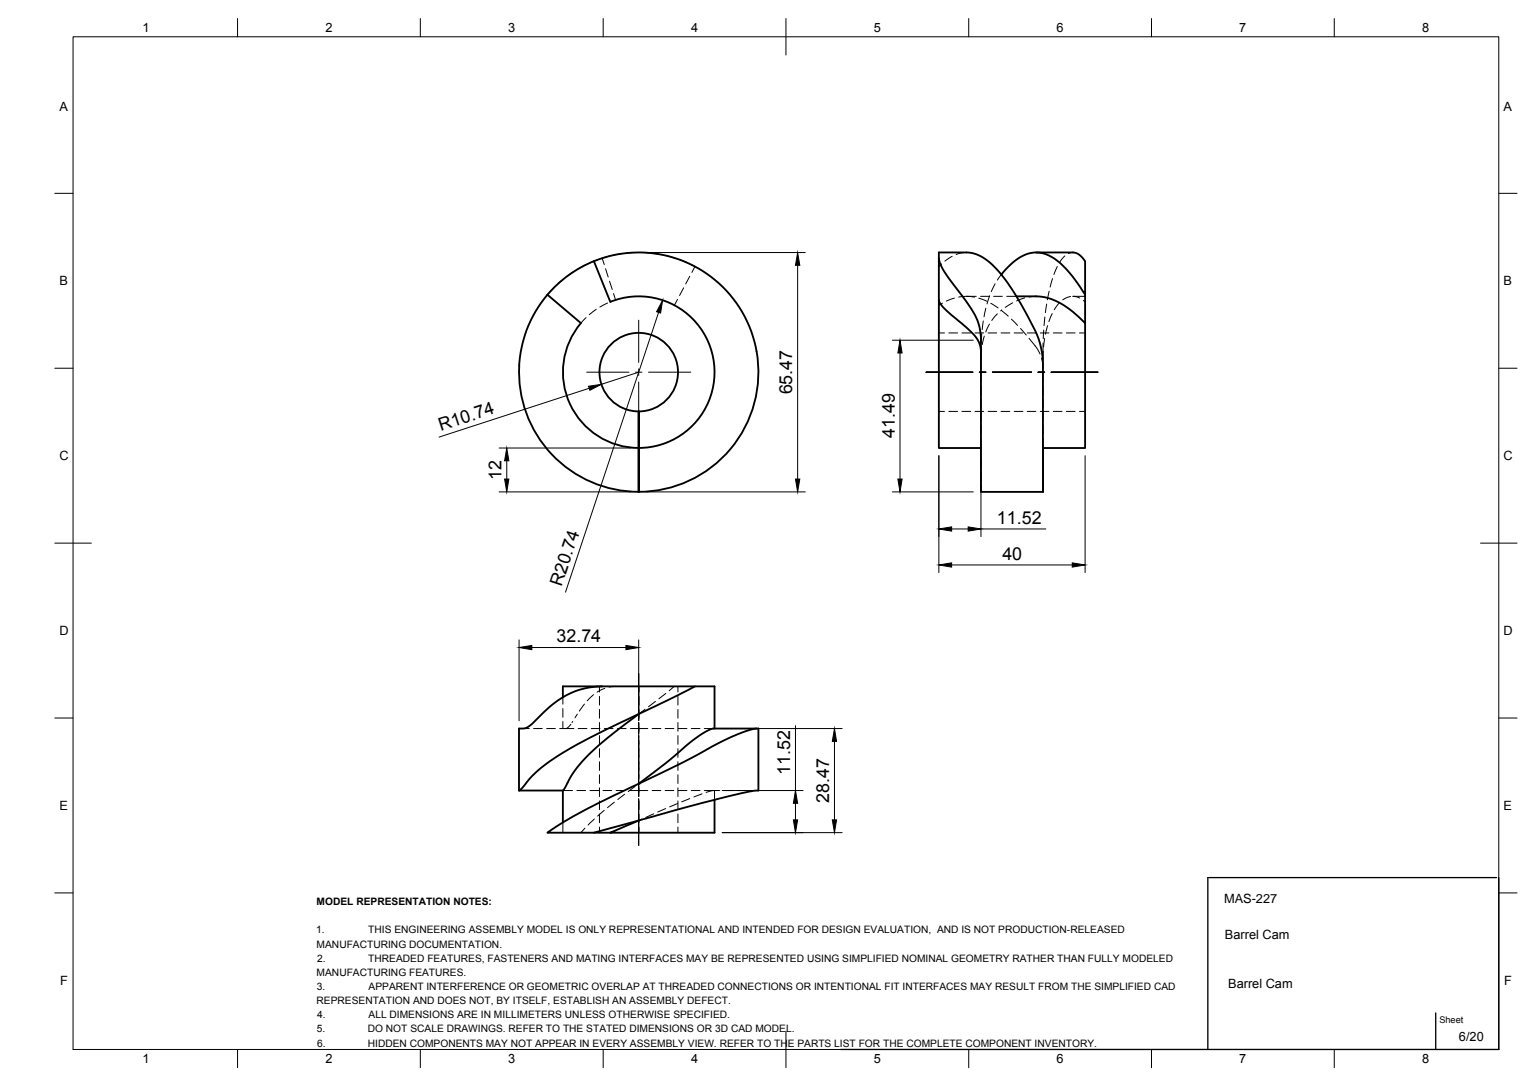
ISO-10303-21;
HEADER;
FILE_DESCRIPTION (('STEP AP214'),
    '1' );
FILE_NAME ( 'Barrel Cam.step', '2026-10-06T08:24:41', ( '' ), ( '' ), 'STEP AP214', 'Unspecified', '' );
FILE_SCHEMA (( 'AUTOMOTIVE_DESIGN' ));
ENDSEC;
DATA;
#20=CARTESIAN_POINT ( 'NONE',  ( 0.3339160553493882300, 0.9180073733179625606, -0.7185233507685039323 ) ) ;
#34=CARTESIAN_POINT ( 'NONE',  ( 0.3976891862754212137, 0.7181140751201200434, -0.6642661073933326943 ) ) ;
#37=ORIENTED_EDGE ( 'NONE', *, *, #10875, .F. ) ;
#42=CARTESIAN_POINT ( 'NONE',  ( -0.3649820351482981340, -1.095990260593795451, -0.3743461065083169559 ) ) ;
#53=DIRECTION ( 'NONE',  ( 0.000000000000000000, 0.000000000000000000, 1.000000000000000000 ) ) ;
#72=CARTESIAN_POINT ( 'NONE',  ( 0.3339160553493882300, 0.7867001919223544082, -0.8344257386302499357 ) ) ;
#75=DIRECTION ( 'NONE',  ( -1.000000000000000000, 0.000000000000000000, 0.000000000000000000 ) ) ;
#104=CARTESIAN_POINT ( 'NONE',  ( -0.6505662911506299162, -0.01797296504513622162, 0.07864818162991654704 ) ) ;
#115=CARTESIAN_POINT ( 'NONE',  ( -0.7432982829791772161, 0.2032415433700952845, -0.2614846436432287091 ) ) ;
#119=CARTESIAN_POINT ( 'NONE',  ( 0.3334645669291338987, -0.9593003268715946108, -0.8847456892490688229 ) ) ;
#171=CARTESIAN_POINT ( 'NONE',  ( -0.3799403784234969272, -1.031940123604548010, -0.2795979895621366063 ) ) ;
#189=ORIENTED_EDGE ( 'NONE', *, *, #329, .F. ) ;
#236=CARTESIAN_POINT ( 'NONE',  ( -0.6370261810203012853, -0.04389326872400071272, -0.2373533611760622331 ) ) ;
#250=CARTESIAN_POINT ( 'NONE',  ( -0.7795729917428700917, 0.3988254141273629982, 0.006455232907575630084 ) ) ;
#260=DIRECTION ( 'NONE',  ( 0.000000000000000000, -0.4702444477782212195, 0.8825362085114445421 ) ) ;
#288=VECTOR ( 'NONE', #25733, 39.37007874015748143 ) ;
#293=CARTESIAN_POINT ( 'NONE',  ( 0.6947676139410623453, 0.7729092381583980709, -0.02125091332446964881 ) ) ;
#329=EDGE_CURVE ( 'NONE', #8378, #18994, #15536, .T. ) ;
#341=B_SPLINE_CURVE_WITH_KNOTS ( 'NONE', 3,
 ( #20281, #13782, #13925, #26772, #18280, #24375, #3448, #26627, #7564, #796, #2888, #16049, #22829 ),
 .UNSPECIFIED., .F., .F.,
 ( 4, 3, 3, 3, 4 ),
 ( 0.01512411120486024073, 0.01814893344583978774, 0.02117375568681436129, 0.02419857792778855668, 0.02712411120487693422 ),
 .UNSPECIFIED. ) ;
#351=CARTESIAN_POINT ( 'NONE',  ( 0.1532705055535415473, -0.8125630895486949390, -0.04838628589907047889 ) ) ;
#357=ORIENTED_EDGE ( 'NONE', *, *, #17696, .F. ) ;
#371=CARTESIAN_POINT ( 'NONE',  ( -0.7635713814939685262, 0.2506761191097937047, -0.2749095812957952911 ) ) ;
#379=CARTESIAN_POINT ( 'NONE',  ( -0.7874015748031496509, 0.8628702403565570167, -0.3208896918748870286 ) ) ;
#411=( GEOMETRIC_REPRESENTATION_CONTEXT ( 3 ) GLOBAL_UNCERTAINTY_ASSIGNED_CONTEXT ( ( #18335 ) ) GLOBAL_UNIT_ASSIGNED_CONTEXT ( ( #27464, #8113, #23091 ) ) REPRESENTATION_CONTEXT ( 'NONE', 'WORKASPACE' ) ) ;
#419=CARTESIAN_POINT ( 'NONE',  ( 0.6015839972843660677, 0.9161431246486984037, -0.1460888818946199375 ) ) ;
#430=DIRECTION ( 'NONE',  ( -1.000000000000000000, 0.000000000000000000, 0.000000000000000000 ) ) ;
#452=CARTESIAN_POINT ( 'NONE',  ( -0.3040421205569480145, 1.249037478091203024, -0.7140903627573721435 ) ) ;
#459=ORIENTED_EDGE ( 'NONE', *, *, #5759, .F. ) ;
#461=DIRECTION ( 'NONE',  ( -1.000000000000000000, 0.000000000000000000, 0.000000000000000000 ) ) ;
#469=CARTESIAN_POINT ( 'NONE',  ( 0.1120675189988346587, -0.7410715175625038897, 0.001857066358701141805 ) ) ;
#483=ADVANCED_FACE ( 'NONE', ( #19377 ), #13015, .T. ) ;
#485=CARTESIAN_POINT ( 'NONE',  ( -0.6370261810203012853, -0.05236013009244417510, -0.08009157605482203346 ) ) ;
#501=CARTESIAN_POINT ( 'NONE',  ( -0.3355349563089153886, 0.1597155962083088576, 0.2362204724409449064 ) ) ;
#527=VERTEX_POINT ( 'NONE', #4408 ) ;
#537=CARTESIAN_POINT ( 'NONE',  ( 0.3843128886798082844, 0.1691648655974895832, -0.07874015748031495954 ) ) ;
#539=CARTESIAN_POINT ( 'NONE',  ( 0.7732217274635454496, 0.5458307047179269400, 0.1151719495065113841 ) ) ;
#550=VERTEX_POINT ( 'NONE', #15439 ) ;
#557=ORIENTED_EDGE ( 'NONE', *, *, #23990, .T. ) ;
#578=EDGE_CURVE ( 'NONE', #17699, #24360, #11458, .T. ) ;
#591=DIRECTION ( 'NONE',  ( 0.000000000000000000, 0.000000000000000000, 1.000000000000000000 ) ) ;
#599=CARTESIAN_POINT ( 'NONE',  ( 0.7872492035923605025, 0.2530564255242896410, -0.2780832379081621952 ) ) ;
#607=VERTEX_POINT ( 'NONE', #866 ) ;
#609=B_SPLINE_CURVE_WITH_KNOTS ( 'NONE', 3,
 ( #16712, #27310, #3855, #5987 ),
 .UNSPECIFIED., .F., .F.,
 ( 4, 4 ),
 ( 0.000000000000000000, 1.000000000000000000 ),
 .UNSPECIFIED. ) ;
#614=APPLICATION_CONTEXT ( 'automotive_design' ) ;
#628=CARTESIAN_POINT ( 'NONE',  ( -0.6633461167951516524, 0.02279600110638677068, 0.07858347093486456325 ) ) ;
#672=CARTESIAN_POINT ( 'NONE',  ( 0.6932508136109228891, 0.7757875710709564165, -0.02341522039927820473 ) ) ;
#686=ORIENTED_EDGE ( 'NONE', *, *, #11935, .F. ) ;
#717=CARTESIAN_POINT ( 'NONE',  ( -0.6562077975700453258, 2.612916929133858441E-14, 0.2362204724409449064 ) ) ;
#736=CARTESIAN_POINT ( 'NONE',  ( 0.7845931698711713365, 0.4599168999537228686, -0.01300178342961078731 ) ) ;
#754=CARTESIAN_POINT ( 'NONE',  ( -0.1259131187103122163, 1.099024551511217362, -0.3668305760060864840 ) ) ;
#796=CARTESIAN_POINT ( 'NONE',  ( 0.7874015748031496509, 0.2841772834048059693, -0.1654443243217737780 ) ) ;
#801=ORIENTED_EDGE ( 'NONE', *, *, #20824, .F. ) ;
#805=CARTESIAN_POINT ( 'NONE',  ( -0.6912180915490531152, 0.1281909420063060967, 0.2299950541617507838 ) ) ;
#824=VECTOR ( 'NONE', #13835, 39.37007874015748143 ) ;
#846=B_SPLINE_CURVE_WITH_KNOTS ( 'NONE', 3,
 ( #20384, #22082, #9633, #24207 ),
 .UNSPECIFIED., .F., .F.,
 ( 4, 4 ),
 ( -1.254364830977226175, -0.8024850953550110022 ),
 .UNSPECIFIED. ) ;
#866=CARTESIAN_POINT ( 'NONE',  ( -0.7874015748031496509, 0.000000000000000000, -0.2362204724409448231 ) ) ;
#921=DIRECTION ( 'NONE',  ( -1.000000000000000000, 0.000000000000000000, 0.000000000000000000 ) ) ;
#927=CARTESIAN_POINT ( 'NONE',  ( -0.7795729917428700917, 0.2877957735339043421, -0.2883818734248744242 ) ) ;
#944=DIRECTION ( 'NONE',  ( -1.000000000000000000, 0.000000000000000000, 0.000000000000000000 ) ) ;
#945=ORIENTED_EDGE ( 'NONE', *, *, #10724, .F. ) ;
#955=CARTESIAN_POINT ( 'NONE',  ( -0.3334645669291338987, 0.9667105296868090392, -0.8968761852611063512 ) ) ;
#957=CARTESIAN_POINT ( 'NONE',  ( 0.7871730179869350641, 0.2557924603611196890, -0.2773276354978094771 ) ) ;
#971=CYLINDRICAL_SURFACE ( 'NONE', #8819, 0.8163976377952756325 ) ;
#999=CARTESIAN_POINT ( 'NONE',  ( -0.6187452617803784749, -0.1345185900882266972, 0.2292394813352827132 ) ) ;
#1009=PLANE ( 'NONE',  #9843 ) ;
#1014=VECTOR ( 'NONE', #23279, 39.37007874015748143 ) ;
#1018=CARTESIAN_POINT ( 'NONE',  ( 0.7874015748031325534, 0.2490515971710990650, -0.2751036149061643621 ) ) ;
#1059=ORIENTED_EDGE ( 'NONE', *, *, #21507, .T. ) ;
#1084=CARTESIAN_POINT ( 'NONE',  ( 0.04115487667019134682, -0.3914832076178914044, -0.3299005569521964443 ) ) ;
#1087=CARTESIAN_POINT ( 'NONE',  ( -0.3607509115914968589, -0.7060833311703261783, -0.6427979834437553830 ) ) ;
#1108=CARTESIAN_POINT ( 'NONE',  ( -0.3453142639840502404, -1.185886736896986315, -0.5421347595288529275 ) ) ;
#1111=CARTESIAN_POINT ( 'NONE',  ( 0.7874015748031496509, -0.6060691875862894706, 0.08482860590294842573 ) ) ;
#1131=CARTESIAN_POINT ( 'NONE',  ( -0.3338887748335582772, -5.862181872598426086E-06, -1.869015748010449007 ) ) ;
#1142=CARTESIAN_POINT ( 'NONE',  ( -0.6119659649693193204, -0.1584167327113908397, 0.2264510984896760670 ) ) ;
#1150=ORIENTED_EDGE ( 'NONE', *, *, #8559, .T. ) ;
#1203=VERTEX_POINT ( 'NONE', #5482 ) ;
#1210=CARTESIAN_POINT ( 'NONE',  ( -0.4473595089310440920, -0.4824549569468952748, -0.3934827063516405654 ) ) ;
#1223=EDGE_CURVE ( 'NONE', #6621, #1203, #26524, .T. ) ;
#1226=CARTESIAN_POINT ( 'NONE',  ( -0.4315274442044927383, -0.5217045752503943756, -0.4246611536723189917 ) ) ;
#1233=CARTESIAN_POINT ( 'NONE',  ( -0.7874015748031496509, 0.4828108945773819105, 0.1423708153504031348 ) ) ;
#1245=CARTESIAN_POINT ( 'NONE',  ( -0.6562077975700374433, -1.365924015748031427E-17, -0.2362204724409449064 ) ) ;
#1286=ORIENTED_EDGE ( 'NONE', *, *, #4049, .F. ) ;
#1295=MECHANICAL_DESIGN_GEOMETRIC_PRESENTATION_REPRESENTATION('',(#17528),#411);
#1296=CARTESIAN_POINT ( 'NONE',  ( 0.3334645669291338987, -9.254566434606299706E-06, -2.341456692880161228 ) ) ;
#1332=CARTESIAN_POINT ( 'NONE',  ( 0.7874015748031496509, -0.3839064563524846596, -0.3321176343386791907 ) ) ;
#1344=CARTESIAN_POINT ( 'NONE',  ( -0.4473595089310440920, -0.5755188248839795406, -0.2663378075042964754 ) ) ;
#1351=CARTESIAN_POINT ( 'NONE',  ( 0.04115487667019118723, -0.4669989807942504512, -0.1904908102188472563 ) ) ;
#1354=CARTESIAN_POINT ( 'NONE',  ( -0.3611843684950729050, -0.7048611138537562715, -0.6407005967225004595 ) ) ;
#1365=CARTESIAN_POINT ( 'NONE',  ( -0.3040421205569480145, 0.7911861580938169825, -0.8381822164908544481 ) ) ;
#1381=EDGE_LOOP ( 'NONE', ( #20318, #13723, #8612, #11698 ) ) ;
#1404=CARTESIAN_POINT ( 'NONE',  ( -0.5969400767949351039, -0.2109524265843517599, 0.2188413833799605912 ) ) ;
#1435=EDGE_CURVE ( 'NONE', #22878, #15456, #5641, .T. ) ;
#1462=CARTESIAN_POINT ( 'NONE',  ( 0.7874015748031496509, -0.5320149438416890142, -0.05415347417759425186 ) ) ;
#1476=ORIENTED_EDGE ( 'NONE', *, *, #20100, .F. ) ;
#1493=CARTESIAN_POINT ( 'NONE',  ( -0.6107239227225801370, -0.1031077391523354814, -0.2427576718125873390 ) ) ;
#1501=CARTESIAN_POINT ( 'NONE',  ( -0.3338887748335570560, -0.8039705855317598182, -0.9107153245080098491 ) ) ;
#1506=CARTESIAN_POINT ( 'NONE',  ( -0.3334645669291338987, 1.129605998290730273, -0.9896751316273187937 ) ) ;
#1514=CARTESIAN_POINT ( 'NONE',  ( -0.8725268807032540153, 0.000000000000000000, 0.2362204724409449619 ) ) ;
#1549=CARTESIAN_POINT ( 'NONE',  ( -0.4168742999989611953, -0.8811754754189499161, -0.1087450224342711852 ) ) ;
#1602=CARTESIAN_POINT ( 'NONE',  ( 0.7874015748031496509, -0.6060691875862913580, 0.08482860590294803715 ) ) ;
#1618=CARTESIAN_POINT ( 'NONE',  ( -0.6002615430280354714, -0.1262890666645074822, -0.2459980689859385949 ) ) ;
#1631=EDGE_LOOP ( 'NONE', ( #23698, #24312, #24788, #16424 ) ) ;
#1632=CARTESIAN_POINT ( 'NONE',  ( -0.6200889942125548115, -0.08218921327254806453, -0.2403616042849680556 ) ) ;
#1652=CARTESIAN_POINT ( 'NONE',  ( -0.3338887748335582772, -9.254566434645669797E-06, -2.341456692880161228 ) ) ;
#1667=ADVANCED_FACE ( 'NONE', ( #18269 ), #10473, .F. ) ;
#1688=CARTESIAN_POINT ( 'NONE',  ( -0.4506204254121950470, -0.7490950376702004698, -0.003669893536069110569 ) ) ;
#1709=CARTESIAN_POINT ( 'NONE',  ( -0.8725268807032540153, 0.000000000000000000, -0.2362204724409448231 ) ) ;
#1754=EDGE_CURVE ( 'NONE', #4466, #3563, #22640, .T. ) ;
#1756=CARTESIAN_POINT ( 'NONE',  ( -0.5546128944410685380, -0.2284628647922791467, -0.2687227238212893665 ) ) ;
#1778=CARTESIAN_POINT ( 'NONE',  ( -0.2602238532265429005, 0.000000000000000000, -0.2362204724409449064 ) ) ;
#1786=EDGE_CURVE ( 'NONE', #3563, #16499, #2562, .T. ) ;
#1796=CARTESIAN_POINT ( 'NONE',  ( -0.7434700980050995556, 0.5844848647591116553, -0.4795863528207047755 ) ) ;
#1800=EDGE_CURVE ( 'NONE', #5887, #6621, #23801, .T. ) ;
#1821=ORIENTED_EDGE ( 'NONE', *, *, #19932, .F. ) ;
#1831=CARTESIAN_POINT ( 'NONE',  ( -0.6054712446264385317, -0.1811734661067123109, 0.2234263948845375547 ) ) ;
#1835=CIRCLE ( 'NONE', #17621, 0.8163976377952757435 ) ;
#1897=ORIENTED_EDGE ( 'NONE', *, *, #23990, .F. ) ;
#1898=CARTESIAN_POINT ( 'NONE',  ( -0.4881018399981850719, -0.4577461864050251794, -0.1927445091220988116 ) ) ;
#1904=B_SPLINE_SURFACE_WITH_KNOTS ( 'NONE', 3, 3, ( 
 ( #4850, #11356, #19838, #9087 ),
 ( #13465, #19569, #6573, #15614 ),
 ( #19703, #17579, #628, #22090 ),
 ( #21544, #17302, #2722, #15199 ),
 ( #15479, #19423, #21823, #24075 ),
 ( #10945, #2458, #26328, #6714 ),
 ( #23810, #2316, #25784, #4580 ),
 ( #4715, #19972, #6991, #15068 ),
 ( #11213, #23678, #11085, #4313 ),
 ( #115, #12918, #2189, #10807 ),
 ( #371, #4452, #8686, #26192 ),
 ( #23944, #6850, #250, #8821 ),
 ( #17437, #11491, #17837, #7390 ) ),
 .UNSPECIFIED., .F., .F., .F.,
 ( 4, 1, 1, 1, 1, 1, 1, 1, 1, 1, 4 ),
 ( 4, 4 ),
 ( 0.3833360769390280476, 0.3893635454205919832, 0.3944867497131970269, 0.4047331582984080023, 0.4098563625910129904, 0.4201027711762239658, 0.4252259754688289539, 0.4405955883466449730, 0.4508419969318550047, 0.4713348141022760118, 0.4911627496483090272 ),
 ( -0.5999999999999999778, 0.5999999999999999778 ),
 .UNSPECIFIED. ) ;
#1915=ORIENTED_EDGE ( 'NONE', *, *, #329, .T. ) ;
#1955=ADVANCED_FACE ( 'NONE', ( #11280 ), #971, .T. ) ;
#1967=CARTESIAN_POINT ( 'NONE',  ( -0.4413253306211258331, -0.7852380862899401848, -0.03056779453504937169 ) ) ;
#1982=ORIENTED_EDGE ( 'NONE', *, *, #10724, .T. ) ;
#1984=CARTESIAN_POINT ( 'NONE',  ( -0.6562077975700374433, -2.731848031496062854E-17, 0.07874015748031495954 ) ) ;
#1990=AXIS2_PLACEMENT_3D ( 'NONE', #5836, #3689, #3843 ) ;
#2001=VECTOR ( 'NONE', #27161, 39.37007874015748143 ) ;
#2012=CARTESIAN_POINT ( 'NONE',  ( 0.3334645669291338987, -9.254566434645669797E-06, -2.341456692880161228 ) ) ;
#2018=VECTOR ( 'NONE', #6496, 39.37007874015748143 ) ;
#2022=CARTESIAN_POINT ( 'NONE',  ( 0.3339160553493882300, 0.7867001919223544082, -0.8344257386302499357 ) ) ;
#2039=CARTESIAN_POINT ( 'NONE',  ( -0.5439522672647024715, -0.3991687350992441097, 0.1730343859005041562 ) ) ;
#2050=B_SPLINE_CURVE_WITH_KNOTS ( 'NONE', 3,
 ( #2022, #4684, #4431, #21940 ),
 .UNSPECIFIED., .F., .F.,
 ( 4, 4 ),
 ( -1.199999999999999956, 0.000000000000000000 ),
 .UNSPECIFIED. ) ;
#2051=CARTESIAN_POINT ( 'NONE',  ( -0.5255103840667624260, -0.2955129232484599577, -0.2915374615789483315 ) ) ;
#2055=CARTESIAN_POINT ( 'NONE',  ( 0.1120675189988346587, -0.4694218845611126678, -0.3846748511993472452 ) ) ;
#2098=ORIENTED_EDGE ( 'NONE', *, *, #19489, .F. ) ;
#2099=CARTESIAN_POINT ( 'NONE',  ( 0.3843128886798082844, 0.1418101685956718039, -0.2362204724398992428 ) ) ;
#2100=CARTESIAN_POINT ( 'NONE',  ( 0.4895462770359960136, 1.042587244177305195, -0.2949132003431567117 ) ) ;
#2142=CARTESIAN_POINT ( 'NONE',  ( 0.3334645669291338987, -0.8041772776331653771, -0.9118913923173522784 ) ) ;
#2158=EDGE_CURVE ( 'NONE', #15240, #27472, #9611, .T. ) ;
#2164=CARTESIAN_POINT ( 'NONE',  ( 0.3334645669291338987, -1.243457723967850148, -0.6813714283177954023 ) ) ;
#2183=CARTESIAN_POINT ( 'NONE',  ( -0.5632721120450597807, -0.3296178001376885436, 0.1935414926636310762 ) ) ;
#2189=CARTESIAN_POINT ( 'NONE',  ( -0.7432982829791772161, 0.2816507422265389637, 0.04372923255535362402 ) ) ;
#2203=AXIS2_PLACEMENT_3D ( 'NONE', #11919, #13750, #9357 ) ;
#2221=CARTESIAN_POINT ( 'NONE',  ( 0.3339160553493882300, 0.9384519710407874804, -0.7923371756411300426 ) ) ;
#2238=DIRECTION ( 'NONE',  ( 0.000000000000000000, 7.180547322999998243E-06, 0.9999999999742198442 ) ) ;
#2263=CARTESIAN_POINT ( 'NONE',  ( 0.3334645669291338987, -5.862181872598426086E-06, -1.869015748010449007 ) ) ;
#2275=DIRECTION ( 'NONE',  ( 0.000000000000000000, 0.000000000000000000, 1.000000000000000000 ) ) ;
#2316=CARTESIAN_POINT ( 'NONE',  ( -0.6996199877990079141, 0.1202923534080998086, -0.08607181623015019989 ) ) ;
#2343=ORIENTED_EDGE ( 'NONE', *, *, #14128, .T. ) ;
#2345=ORIENTED_EDGE ( 'NONE', *, *, #4798, .T. ) ;
#2362=FACE_OUTER_BOUND ( 'NONE', #12318, .T. ) ;
#2365=CARTESIAN_POINT ( 'NONE',  ( 0.7107691196319370075, 0.7407165212924035069, 0.002142197690853237663 ) ) ;
#2383=EDGE_LOOP ( 'NONE', ( #2870, #1150, #13104, #24041 ) ) ;
#2451=ORIENTED_EDGE ( 'NONE', *, *, #17265, .T. ) ;
#2458=CARTESIAN_POINT ( 'NONE',  ( -0.6912180915490531152, 0.09686421027289587871, -0.08344423162361633284 ) ) ;
#2462=FACE_OUTER_BOUND ( 'NONE', #13499, .T. ) ;
#2471=LINE ( 'NONE', #4590, #14912 ) ;
#2491=ORIENTED_EDGE ( 'NONE', *, *, #5759, .T. ) ;
#2493=DIRECTION ( 'NONE',  ( -1.000000000000000000, 0.000000000000000000, 0.000000000000000000 ) ) ;
#2506=CARTESIAN_POINT ( 'NONE',  ( 0.3976891862754212137, 0.9951575781684135480, -0.5144425584461574941 ) ) ;
#2508=CARTESIAN_POINT ( 'NONE',  ( 0.7838584557816548060, 0.4717991116846240174, 0.1472977909967729537 ) ) ;
#2562=B_SPLINE_CURVE_WITH_KNOTS ( 'NONE', 3,
 ( #5700, #12044, #18522, #14313 ),
 .UNSPECIFIED., .F., .F.,
 ( 4, 4 ),
 ( 0.000000000000000000, 0.4421524820080139917 ),
 .UNSPECIFIED. ) ;
#2578=CARTESIAN_POINT ( 'NONE',  ( -0.6305589872448129629, -0.06986321629937303213, -0.08121850359745433345 ) ) ;
#2596=CARTESIAN_POINT ( 'NONE',  ( -0.6869867706933208140, 0.7419671345971732279, -0.1783180911161240390 ) ) ;
#2672=DIRECTION ( 'NONE',  ( 0.000000000000000000, -0.5749917231862786693, 0.8181592254978695689 ) ) ;
#2690=CARTESIAN_POINT ( 'NONE',  ( 0.1120675189988346587, -0.4694218845611126678, -0.3846748511993476338 ) ) ;
#2692=CARTESIAN_POINT ( 'NONE',  ( 0.7430739993161732393, 0.4432762660064943905, -0.3627962913661458288 ) ) ;
#2706=DIRECTION ( 'NONE',  ( -1.000000000000000000, 0.000000000000000000, 0.000000000000000000 ) ) ;
#2711=CARTESIAN_POINT ( 'NONE',  ( -0.6262477747318130339, -0.09467419725595611901, 0.07480744568936535666 ) ) ;
#2713=EDGE_CURVE ( 'NONE', #15744, #16084, #3962, .T. ) ;
#2722=CARTESIAN_POINT ( 'NONE',  ( -0.6722178168900768691, 0.05124196228576535783, 0.07772299437287735757 ) ) ;
#2726=ORIENTED_EDGE ( 'NONE', *, *, #25744, .T. ) ;
#2731=CARTESIAN_POINT ( 'NONE',  ( -0.3355349563089150000, 0.1402003033445870239, 0.07874015748031495954 ) ) ;
#2739=AXIS2_PLACEMENT_3D ( 'NONE', #23817, #4184, #16905 ) ;
#2761=ORIENTED_EDGE ( 'NONE', *, *, #2947, .F. ) ;
#2765=CARTESIAN_POINT ( 'NONE',  ( -0.03794311743615354227, 0.6358669483106004217, -0.5146366652951276377 ) ) ;
#2824=CARTESIAN_POINT ( 'NONE',  ( 0.7871730179869745880, 0.2548056305271102495, -0.2803186531705669227 ) ) ;
#2844=CARTESIAN_POINT ( 'NONE',  ( -0.6370261810203012853, -0.06929385342672342296, 0.2344319926069744209 ) ) ;
#2867=DIRECTION ( 'NONE',  ( 0.000000000000000000, -7.180547322999995702E-06, -0.9999999999742197332 ) ) ;
#2870=ORIENTED_EDGE ( 'NONE', *, *, #10426, .F. ) ;
#2888=CARTESIAN_POINT ( 'NONE',  ( 0.7874015748031496509, 0.2724655384146937864, -0.2020072023942773021 ) ) ;
#2892=ORIENTED_EDGE ( 'NONE', *, *, #1435, .F. ) ;
#2924=CARTESIAN_POINT ( 'NONE',  ( 0.3339160553493877859, 5.862181872598426086E-06, -1.869015748010449007 ) ) ;
#2947=EDGE_CURVE ( 'NONE', #24281, #22748, #24233, .T. ) ;
#2953=CARTESIAN_POINT ( 'NONE',  ( 0.3339160553493882300, 0.000000000000000000, -1.052618110236220428 ) ) ;
#2965=CARTESIAN_POINT ( 'NONE',  ( 0.7430739993161732393, 0.6166684212952147082, -0.09296748371178542580 ) ) ;
#2984=CARTESIAN_POINT ( 'NONE',  ( 0.3667188884249754643, 0.2611681335937625636, 0.2162202218317502145 ) ) ;
#3010=CARTESIAN_POINT ( 'NONE',  ( -0.7246715730664488042, 0.1595564285404119931, -0.2516711161248811335 ) ) ;
#3011=ORIENTED_EDGE ( 'NONE', *, *, #578, .F. ) ;
#3014=CARTESIAN_POINT ( 'NONE',  ( -0.3503688343903059166, -1.161116239014858387, -0.4867237306978748346 ) ) ;
#3037=CARTESIAN_POINT ( 'NONE',  ( 0.3843128886798082844, 0.2238742596014886010, 0.2362204724409449064 ) ) ;
#3049=CARTESIAN_POINT ( 'NONE',  ( -0.3338887748335570005, -1.256685249340607546, -0.7575795143361759854 ) ) ;
#3106=ADVANCED_FACE ( 'NONE', ( #26499 ), #24657, .T. ) ;
#3112=CARTESIAN_POINT ( 'NONE',  ( 0.7430739993161732393, 0.4424178910903722728, -0.3641321082570454504 ) ) ;
#3161=CARTESIAN_POINT ( 'NONE',  ( -0.3338887748335567229, -1.257773430019720307, -0.7637447580504644895 ) ) ;
#3174=CARTESIAN_POINT ( 'NONE',  ( -0.3558329076891611487, -0.7201416780480096591, -0.6679878162024859289 ) ) ;
#3235=CARTESIAN_POINT ( 'NONE',  ( -0.8725268807032540153, 0.000000000000000000, -1.052618110236220428 ) ) ;
#3243=CARTESIAN_POINT ( 'NONE',  ( 0.4895462770358314786, 1.042587244177472394, -0.2949132003433866389 ) ) ;
#3300=CARTESIAN_POINT ( 'NONE',  ( -0.4280150452258433269, -0.8372280483532893447, -0.07105027534967854608 ) ) ;
#3308=CARTESIAN_POINT ( 'NONE',  ( -0.2602238532265429005, 0.000000000000000000, -0.07874015748031495954 ) ) ;
#3311=CARTESIAN_POINT ( 'NONE',  ( -0.4300685960020619314, -0.5253395418799321481, -0.4276959590273259337 ) ) ;
#3322=CARTESIAN_POINT ( 'NONE',  ( 0.5885985490145342336, 0.9326256249715371149, -0.1629194618731351907 ) ) ;
#3344=CARTESIAN_POINT ( 'NONE',  ( 0.3334645669291338987, -1.269546425348450747, -0.8304542831125020230 ) ) ;
#3396=MANIFOLD_SOLID_BREP ( 'Barrel Cam', #16864 ) ;
#3438=CARTESIAN_POINT ( 'NONE',  ( -0.3376790527244098450, -1.075350501301808981, -0.6872880233270275419 ) ) ;
#3448=CARTESIAN_POINT ( 'NONE',  ( 0.7874015748031496509, 0.3205050385779313893, -0.05203301786850960536 ) ) ;
#3452=EDGE_CURVE ( 'NONE', #10641, #13674, #10781, .T. ) ;
#3476=AXIS2_PLACEMENT_3D ( 'NONE', #15362, #6861, #260 ) ;
#3481=CARTESIAN_POINT ( 'NONE',  ( 0.5394643376411901725, -0.1051622988770984091, 0.2362204724409454060 ) ) ;
#3509=CARTESIAN_POINT ( 'NONE',  ( -0.6091215340374328546, -0.1684002209738235112, 0.2251732882052777107 ) ) ;
#3531=DIRECTION ( 'NONE',  ( 0.000000000000000000, 0.000000000000000000, 1.000000000000000000 ) ) ;
#3563=VERTEX_POINT ( 'NONE', #18687 ) ;
#3578=ORIENTED_EDGE ( 'NONE', *, *, #25897, .F. ) ;
#3598=CARTESIAN_POINT ( 'NONE',  ( -0.4958319195689224190, -0.3652762862495049223, -0.3220933753858993831 ) ) ;
#3636=AXIS2_PLACEMENT_3D ( 'NONE', #19978, #11362, #24351 ) ;
#3655=CARTESIAN_POINT ( 'NONE',  ( -0.5347915442629350702, -0.4325403863649552871, 0.1614721600616167985 ) ) ;
#3658=CARTESIAN_POINT ( 'NONE',  ( -0.7874015748031496509, -5.862181872755905604E-06, -1.869015748010449007 ) ) ;
#3665=DIRECTION ( 'NONE',  ( 0.000000000000000000, 0.000000000000000000, 1.000000000000000000 ) ) ;
#3678=DIRECTION ( 'NONE',  ( -1.000000000000000000, 0.000000000000000000, 0.000000000000000000 ) ) ;
#3689=DIRECTION ( 'NONE',  ( -1.000000000000000000, 0.000000000000000000, 0.000000000000000000 ) ) ;
#3717=FACE_OUTER_BOUND ( 'NONE', #1381, .T. ) ;
#3724=AXIS2_PLACEMENT_3D ( 'NONE', #6641, #430, #17889 ) ;
#3730=VERTEX_POINT ( 'NONE', #20649 ) ;
#3733=CARTESIAN_POINT ( 'NONE',  ( -0.5935113537020059171, -0.1411927790378836589, -0.2484461867309594729 ) ) ;
#3745=ORIENTED_EDGE ( 'NONE', *, *, #10571, .T. ) ;
#3748=CARTESIAN_POINT ( 'NONE',  ( -0.5738238537687410101, -0.1850264159751985327, -0.2573737795900459813 ) ) ;
#3776=LINE ( 'NONE', #21010, #14306 ) ;
#3777=B_SPLINE_CURVE_WITH_KNOTS ( 'NONE', 3,
 ( #20017, #13247, #2508, #8735, #539, #23867, #11127, #4500, #25974, #9130, #24390, #13381, #17624, #6627, #17749, #2365, #4901, #15655, #19623, #293, #24255, #8866, #11398, #672, #17487, #9262, #26107, #6764, #19750, #15397, #23989, #419, #26240, #6898, #7583, #20434, #3322, #9401, #25091, #11675, #11964, #9697, #20584, #16208, #15917 ),
 .UNSPECIFIED., .F., .F.,
 ( 4, 2, 1, 1, 1, 1, 2, 2, 2, 2, 1, 1, 1, 1, 1, 2, 2, 2, 2, 1, 1, 1, 1, 2, 2, 2, 2, 2, 4 ),
 ( 0.000000000000000000, 0.1250000000000077716, 0.1875000000000116018, 0.2187500000000134892, 0.2343750000000144607, 0.2421875000000147937, 0.2460937500000149880, 0.2500000000000151545, 0.3750000000000195399, 0.4375000000000214273, 0.4687500000000222045, 0.4843750000000223710, 0.4921875000000224820, 0.4960937500000226485, 0.4980468750000229816, 0.4990234375000230371, 0.5000000000000230926, 0.6250000000000341949, 0.6875000000000397460, 0.7187500000000424105, 0.7343750000000437428, 0.7421875000000444089, 0.7460937500000445199, 0.7480468750000444089, 0.7500000000000442979, 0.8125000000000331957, 0.8437500000000276446, 0.8750000000000222045, 1.000000000000000000 ),
 .UNSPECIFIED. ) ;
#3785=CARTESIAN_POINT ( 'NONE',  ( 0.7873254110137047901, 0.3967163408419193127, 0.1736506122128708696 ) ) ;
#3786=CARTESIAN_POINT ( 'NONE',  ( 0.3339160553493877304, 0.7781263166395089304, -0.8035123328091101635 ) ) ;
#3811=CARTESIAN_POINT ( 'NONE',  ( -0.4339437742824454047, -0.8141188606247102832, -0.05345644696679699437 ) ) ;
#3830=CYLINDRICAL_SURFACE ( 'NONE', #10908, 1.288838582677165556 ) ;
#3843=DIRECTION ( 'NONE',  ( 0.000000000000000000, 0.3746092808414298592, 0.9271827687718677824 ) ) ;
#3855=CARTESIAN_POINT ( 'NONE',  ( 0.3561571326799479742, 1.175382753584212514, -0.5166459152402519406 ) ) ;
#3859=CARTESIAN_POINT ( 'NONE',  ( 0.7874015748031496509, -5.862181872598426086E-06, -1.869015748010449007 ) ) ;
#3881=CARTESIAN_POINT ( 'NONE',  ( -0.5072939182192724994, -0.4034160323192637621, -0.1660794105494917405 ) ) ;
#3893=CARTESIAN_POINT ( 'NONE',  ( -0.4457380174055288191, -0.4863213126542877962, -0.3953166246891253732 ) ) ;
#3908=CARTESIAN_POINT ( 'NONE',  ( 0.5309636003393858328, 0.6336838567619331730, -0.5358812336713733027 ) ) ;
#3954=CARTESIAN_POINT ( 'NONE',  ( -0.5585908902305192214, -0.3463899499700468509, 0.1889404979411018481 ) ) ;
#3962=CIRCLE ( 'NONE', #3476, 0.8163976377952752994 ) ;
#3967=DIRECTION ( 'NONE',  ( -1.000000000000000000, 0.000000000000000000, 0.000000000000000000 ) ) ;
#4004=DIRECTION ( 'NONE',  ( -1.000000000000000000, 0.000000000000000000, 0.000000000000000000 ) ) ;
#4022=CARTESIAN_POINT ( 'NONE',  ( -0.3334645669291338987, 1.286842404713327115, -0.9809137335991812146 ) ) ;
#4026=CARTESIAN_POINT ( 'NONE',  ( -0.5252801253069795395, -0.3531373716088681003, -0.1448790496363011882 ) ) ;
#4041=CARTESIAN_POINT ( 'NONE',  ( -0.6260402177881045915, -0.06877927659531429816, -0.2391228434390870461 ) ) ;
#4049=EDGE_CURVE ( 'NONE', #26227, #527, #10674, .T. ) ;
#4063=CARTESIAN_POINT ( 'NONE',  ( -0.4798812372167961526, 0.2895448272006467261, -0.2870126340407198606 ) ) ;
#4074=CARTESIAN_POINT ( 'NONE',  ( 0.3339160553493882300, 1.066403253539521589, -0.6645352095345236076 ) ) ;
#4094=CARTESIAN_POINT ( 'NONE',  ( -0.4328487442495566051, -0.8184178445223569964, -0.05697890223968492956 ) ) ;
#4165=CARTESIAN_POINT ( 'NONE',  ( -0.4881018399981850719, -0.6057852840965571861, 0.08534609957935157531 ) ) ;
#4168=ORIENTED_EDGE ( 'NONE', *, *, #15874, .T. ) ;
#4180=CARTESIAN_POINT ( 'NONE',  ( -0.6467180715673140901, -0.02183847761193024803, -0.2362204724409446288 ) ) ;
#4184=DIRECTION ( 'NONE',  ( 1.000000000000000000, 0.000000000000000000, 0.000000000000000000 ) ) ;
#4210=ORIENTED_EDGE ( 'NONE', *, *, #19484, .T. ) ;
#4220=ORIENTED_EDGE ( 'NONE', *, *, #19484, .F. ) ;
#4236=CARTESIAN_POINT ( 'NONE',  ( -0.3854046260861516138, -1.009161588507168972, -0.2500462002441404263 ) ) ;
#4244=CARTESIAN_POINT ( 'NONE',  ( -0.7874015748031496509, 0.3058301319751310920, -0.2956682880063846164 ) ) ;
#4251=CARTESIAN_POINT ( 'NONE',  ( -0.6562077975700374433, -2.731848031496062854E-17, -0.1574803149606299191 ) ) ;
#4286=CARTESIAN_POINT ( 'NONE',  ( 0.05001895696127157259, -0.4012255422357954848, -0.3367473437330908426 ) ) ;
#4303=CARTESIAN_POINT ( 'NONE',  ( -0.4995226175161708859, -0.4941169763608158072, -0.03469573555946992016 ) ) ;
#4313=CARTESIAN_POINT ( 'NONE',  ( -0.7246715730664488042, 0.2518900982766236196, 0.2118286996268641809 ) ) ;
#4318=EDGE_CURVE ( 'NONE', #26847, #26227, #22855, .T. ) ;
#4321=CARTESIAN_POINT ( 'NONE',  ( -0.6869867706933208140, 0.5354097223591692822, -0.4217158658263621684 ) ) ;
#4408=CARTESIAN_POINT ( 'NONE',  ( -0.3338887748335570560, -1.269220122646561588, -0.8285976369166339062 ) ) ;
#4414=ORIENTED_EDGE ( 'NONE', *, *, #5878, .F. ) ;
#4431=CARTESIAN_POINT ( 'NONE',  ( 0.3339160553493882300, 1.090203750159222551, -0.7502486126520099274 ) ) ;
#4452=CARTESIAN_POINT ( 'NONE',  ( -0.7635713814939685262, 0.2990306848552756191, -0.1248922643827116152 ) ) ;
#4456=CARTESIAN_POINT ( 'NONE',  ( 0.2249706821157846648, -0.9514344361775100012, -0.1680475531490076835 ) ) ;
#4466=VERTEX_POINT ( 'NONE', #15179 ) ;
#4496=ORIENTED_EDGE ( 'NONE', *, *, #7820, .F. ) ;
#4500=CARTESIAN_POINT ( 'NONE',  ( 0.7623981986069212624, 0.5947989165269446099, 0.09076627200198640610 ) ) ;
#4501=VERTEX_POINT ( 'NONE', #21527 ) ;
#4511=FACE_OUTER_BOUND ( 'NONE', #20713, .T. ) ;
#4515=CYLINDRICAL_SURFACE ( 'NONE', #3724, 1.288838582677165556 ) ;
#4524=PLANE ( 'NONE',  #26001 ) ;
#4569=CARTESIAN_POINT ( 'NONE',  ( -0.6434710025615986151, -0.02921435793731240460, -0.2366737192061291462 ) ) ;
#4578=PLANE ( 'NONE',  #10029 ) ;
#4580=CARTESIAN_POINT ( 'NONE',  ( -0.6996199877990079141, 0.1591959485999228652, 0.2265176967194976465 ) ) ;
#4586=CARTESIAN_POINT ( 'NONE',  ( -0.7874015748031496509, 0.6226544199590670070, -0.5245967315940827103 ) ) ;
#4590=CARTESIAN_POINT ( 'NONE',  ( -0.2602238532265429005, 0.000000000000000000, 0.2362204724409449064 ) ) ;
#4616=B_SPLINE_CURVE_WITH_KNOTS ( 'NONE', 3,
 ( #12687, #12828, #21461, #6761, #2099, #19327 ),
 .UNSPECIFIED., .F., .F.,
 ( 4, 1, 1, 4 ),
 ( 0.000000000000000000, 0.2857142857142853098, 0.5714285714285706197, 1.000000000000000000 ),
 .UNSPECIFIED. ) ;
#4621=CARTESIAN_POINT ( 'NONE',  ( 0.4245040230929275626, 0.9715221028222027488, -0.4707374946848913444 ) ) ;
#4634=DIRECTION ( 'NONE',  ( 0.000000000000000000, 0.000000000000000000, 1.000000000000000000 ) ) ;
#4643=VECTOR ( 'NONE', #21062, 39.37007874015748143 ) ;
#4684=CARTESIAN_POINT ( 'NONE',  ( 0.3339160553493882300, 0.9384519710407874804, -0.7923371756411300426 ) ) ;
#4701=CARTESIAN_POINT ( 'NONE',  ( -0.6112138326843681302, -0.1217116465605828785, -0.08634548179755788255 ) ) ;
#4715=CARTESIAN_POINT ( 'NONE',  ( -0.7121770198535963825, 0.1302456093167436990, -0.2464793285356193242 ) ) ;
#4772=CIRCLE ( 'NONE', #12909, 0.4226968503937005295 ) ;
#4798=EDGE_CURVE ( 'NONE', #25818, #23475, #22481, .T. ) ;
#4816=B_SPLINE_CURVE_WITH_KNOTS ( 'NONE', 3,
 ( #27616, #452, #8258, #4022 ),
 .UNSPECIFIED., .F., .F.,
 ( 4, 4 ),
 ( 0.000000000000000000, 1.000000000000000000 ),
 .UNSPECIFIED. ) ;
#4820=CARTESIAN_POINT ( 'NONE',  ( 0.5309636003393858328, 0.8781547594069606388, -0.3365259449620598975 ) ) ;
#4850=CARTESIAN_POINT ( 'NONE',  ( -0.6562077975700097987, -6.248834645669291056E-14, -0.2362204724409449064 ) ) ;
#4898=FACE_OUTER_BOUND ( 'NONE', #11957, .T. ) ;
#4901=CARTESIAN_POINT ( 'NONE',  ( 0.7057179476745132352, 0.7513714478760473714, -0.005393721693867387784 ) ) ;
#4963=CARTESIAN_POINT ( 'NONE',  ( 0.7871730179869745880, 0.2543122156106876197, -0.2818141620071378251 ) ) ;
#4979=CARTESIAN_POINT ( 'NONE',  ( -0.6112138326843681302, -0.1610742544855759961, 0.2261555117611102339 ) ) ;
#4995=EDGE_CURVE ( 'NONE', #550, #15456, #17942, .T. ) ;
#5006=CIRCLE ( 'NONE', #5947, 1.288838582677165556 ) ;
#5042=CARTESIAN_POINT ( 'NONE',  ( 0.7874015748031496509, 1.344047637795275569E-32, 0.2362204724409449064 ) ) ;
#5094=CARTESIAN_POINT ( 'NONE',  ( 0.6175000359513720394, 0.5724198758948899624, -0.4671145582681361375 ) ) ;
#5106=VECTOR ( 'NONE', #7203, 39.37007874015748854 ) ;
#5113=CARTESIAN_POINT ( 'NONE',  ( 0.4898768902087983768, 0.000000000000000000, 0.2362204724409449064 ) ) ;
#5160=ORIENTED_EDGE ( 'NONE', *, *, #25897, .T. ) ;
#5161=CARTESIAN_POINT ( 'NONE',  ( -0.3969055948396000288, -0.6093040995678481453, -0.5087267836413271738 ) ) ;
#5170=CARTESIAN_POINT ( 'NONE',  ( -0.03794311743615354227, 0.7585235100853641166, -0.4108618826768283827 ) ) ;
#5217=ORIENTED_EDGE ( 'NONE', *, *, #25937, .T. ) ;
#5222=CARTESIAN_POINT ( 'NONE',  ( -0.6226845887534185886, -0.1205360030604272631, 0.2306066678346231080 ) ) ;
#5229=CARTESIAN_POINT ( 'NONE',  ( 0.000000000000000000, 0.000000000000000000, 0.000000000000000000 ) ) ;
#5242=CARTESIAN_POINT ( 'NONE',  ( 0.7874015748031325534, 0.3451340551350263741, 0.02485503895194105320 ) ) ;
#5279=CARTESIAN_POINT ( 'NONE',  ( -0.7874015748031496509, 0.7427623301578110127, -0.4227432117344842588 ) ) ;
#5289=B_SPLINE_CURVE_WITH_KNOTS ( 'NONE', 3,
 ( #27178, #13745, #7819, #5559 ),
 .UNSPECIFIED., .F., .F.,
 ( 4, 4 ),
 ( 0.000000000000000000, 1.199999999999999956 ),
 .UNSPECIFIED. ) ;
#5295=CARTESIAN_POINT ( 'NONE',  ( -0.4280150452258433269, -0.5303309585532346437, -0.4308570359575180642 ) ) ;
#5311=CARTESIAN_POINT ( 'NONE',  ( -0.8725268807032540153, 0.000000000000000000, -1.052618110236220428 ) ) ;
#5332=CARTESIAN_POINT ( 'NONE',  ( 0.6882266799383700562, -0.2663285262597259728, -0.2694682288251842861 ) ) ;
#5333=CARTESIAN_POINT ( 'NONE',  ( -0.3338887748335570560, -1.269220122646561588, -0.8285976369166339062 ) ) ;
#5360=CARTESIAN_POINT ( 'NONE',  ( -0.6116756676109479374, 0.7064581683589515881, 0.02937168582378947568 ) ) ;
#5384=DIRECTION ( 'NONE',  ( 0.000000000000000000, 0.000000000000000000, 1.000000000000000000 ) ) ;
#5393=CARTESIAN_POINT ( 'NONE',  ( 0.7871730179869745880, 0.4038169352867496120, 0.1713250154738354125 ) ) ;
#5402=CARTESIAN_POINT ( 'NONE',  ( -0.3338887748335582772, -9.254566434370079157E-06, -2.341456692880161228 ) ) ;
#5406=ORIENTED_EDGE ( 'NONE', *, *, #22612, .T. ) ;
#5432=B_SPLINE_CURVE_WITH_KNOTS ( 'NONE', 3,
 ( #957, #10251, #17186, #16914, #3908, #21143 ),
 .UNSPECIFIED., .F., .F.,
 ( 4, 1, 1, 4 ),
 ( 0.000000000000000000, 0.4285714285714292138, 0.7142857142857154118, 1.000000000000000000 ),
 .UNSPECIFIED. ) ;
#5445=CARTESIAN_POINT ( 'NONE',  ( -0.7635713814939685262, 0.2506761191097937047, -0.2749095812957952911 ) ) ;
#5447=ORIENTED_EDGE ( 'NONE', *, *, #15874, .F. ) ;
#5448=CARTESIAN_POINT ( 'NONE',  ( -0.3503688343903059166, -1.019241955546190903, -0.5558691273266149757 ) ) ;
#5463=CARTESIAN_POINT ( 'NONE',  ( -0.6806799598997224088, 0.08941145402117105234, 0.2332800728132976564 ) ) ;
#5466=CARTESIAN_POINT ( 'NONE',  ( -0.2490711204941342405, 1.060861271878683176, -0.6594961294738858060 ) ) ;
#5469=FACE_OUTER_BOUND ( 'NONE', #13610, .T. ) ;
#5482=CARTESIAN_POINT ( 'NONE',  ( 0.7874015748031496509, -0.6060691875862894706, 0.08482860590294842573 ) ) ;
#5502=ORIENTED_EDGE ( 'NONE', *, *, #1800, .F. ) ;
#5508=CARTESIAN_POINT ( 'NONE',  ( -0.4798812372167962081, 0.4571014508549643973, 0.1560354075451796108 ) ) ;
#5520=ORIENTED_EDGE ( 'NONE', *, *, #2947, .T. ) ;
#5537=CARTESIAN_POINT ( 'NONE',  ( 0.7871730179869350641, 0.2557924603611196890, -0.2773276354978094771 ) ) ;
#5559=CARTESIAN_POINT ( 'NONE',  ( 0.3976891862754212137, 0.7181140751201200434, -0.6642661073933326943 ) ) ;
#5564=B_SPLINE_CURVE_WITH_KNOTS ( 'NONE', 3,
 ( #9552, #11972, #5332, #24395 ),
 .UNSPECIFIED., .F., .F.,
 ( 4, 4 ),
 ( 0.000000000000000000, 1.000000000000000000 ),
 .UNSPECIFIED. ) ;
#5568=CARTESIAN_POINT ( 'NONE',  ( -0.7874015748031496509, 0.3943205132762559462, -0.07664873632799094894 ) ) ;
#5599=VERTEX_POINT ( 'NONE', #1245 ) ;
#5610=CARTESIAN_POINT ( 'NONE',  ( -0.3334645669291338987, 1.279353152430305007, -0.8465078874097147210 ) ) ;
#5632=CARTESIAN_POINT ( 'NONE',  ( -0.7874015748031496509, 0.4238173070432976197, -0.003642219101859566713 ) ) ;
#5641=B_SPLINE_CURVE_WITH_KNOTS ( 'NONE', 3,
 ( #6324, #1796, #19023, #27658, #8307, #4063, #12668, #21296, #23567, #12807 ),
 .UNSPECIFIED., .F., .F.,
 ( 4, 2, 2, 2, 4 ),
 ( 0.000000000000000000, 0.2500000000000001665, 0.5000000000000001110, 0.7500000000000000000, 1.000000000000000000 ),
 .UNSPECIFIED. ) ;
#5657=CARTESIAN_POINT ( 'NONE',  ( -0.5945615373477443066, -0.2192526351142929930, 0.2174344697355220513 ) ) ;
#5700=CARTESIAN_POINT ( 'NONE',  ( 0.4895462770359960136, 0.6604130065487362478, -0.5726600247964968027 ) ) ;
#5716=CARTESIAN_POINT ( 'NONE',  ( 0.6882266799383700562, -0.3690762517716402180, 0.03266564387697358518 ) ) ;
#5747=CARTESIAN_POINT ( 'NONE',  ( -0.4032359719620975946, -0.5930303427490664081, -0.4910027445640789412 ) ) ;
#5754=DIRECTION ( 'NONE',  ( -1.000000000000000000, 0.000000000000000000, 0.000000000000000000 ) ) ;
#5758=CARTESIAN_POINT ( 'NONE',  ( -0.3334645669291338987, 1.123031841058557134, -0.8716920363354115908 ) ) ;
#5759=EDGE_CURVE ( 'NONE', #26083, #24281, #23468, .T. ) ;
#5761=DIRECTION ( 'NONE',  ( 1.000000000000000000, 0.000000000000000000, 0.000000000000000000 ) ) ;
#5778=CARTESIAN_POINT ( 'NONE',  ( -0.7874015748031496509, 0.4533141008103401259, 0.06936429812427165331 ) ) ;
#5801=CARTESIAN_POINT ( 'NONE',  ( -0.5642276165568446133, -0.3262508299432601011, 0.1942441824117969729 ) ) ;
#5836=CARTESIAN_POINT ( 'NONE',  ( -0.7874015748031496509, 0.000000000000000000, -1.052618110236220428 ) ) ;
#5857=CARTESIAN_POINT ( 'NONE',  ( 0.6882266799383700562, -0.4204501145275968965, 0.1837325802280523612 ) ) ;
#5859=LENGTH_MEASURE_WITH_UNIT ( LENGTH_MEASURE( 0.02539999999999999897 ), #25193 ) ;
#5873=CARTESIAN_POINT ( 'NONE',  ( -0.5743180011325290657, -0.2903071062613433173, 0.2032833715572389954 ) ) ;
#5878=EDGE_CURVE ( 'NONE', #5599, #22369, #23402, .T. ) ;
#5884=CARTESIAN_POINT ( 'NONE',  ( 0.1120675189988346587, -0.6505216398953739265, -0.1269869061606484217 ) ) ;
#5887=VERTEX_POINT ( 'NONE', #25494 ) ;
#5889=CARTESIAN_POINT ( 'NONE',  ( -0.6128263037575037986, -0.09844888684487719532, -0.2421684138024215449 ) ) ;
#5891=CARTESIAN_POINT ( 'NONE',  ( -0.3334645669291338987, 1.286842404713327115, -0.9809137335991812146 ) ) ;
#5942=CARTESIAN_POINT ( 'NONE',  ( -0.4958728716544008042, -0.5762407295275912000, 0.1026277124767580040 ) ) ;
#5947=AXIS2_PLACEMENT_3D ( 'NONE', #19913, #11564, #22306 ) ;
#5966=LINE ( 'NONE', #1709, #21798 ) ;
#5987=CARTESIAN_POINT ( 'NONE',  ( 0.3976891862754212137, 1.133679329692560245, -0.4395307839725697274 ) ) ;
#6010=CARTESIAN_POINT ( 'NONE',  ( -0.5072939182192724994, -0.4686501608227520155, -0.02272223917426736267 ) ) ;
#6025=CARTESIAN_POINT ( 'NONE',  ( -0.6257187983968769407, -0.06950490751670782008, -0.2391845094378674264 ) ) ;
#6063=CARTESIAN_POINT ( 'NONE',  ( 0.3561571326799479742, 0.8881672886669704781, -0.6476052193426063974 ) ) ;
#6087=CARTESIAN_POINT ( 'NONE',  ( -0.6097469662162354753, -0.1662068818069558362, 0.2254586359451796196 ) ) ;
#6149=PRESENTATION_STYLE_ASSIGNMENT (( #21387 ) ) ;
#6164=CARTESIAN_POINT ( 'NONE',  ( -0.4609540795476803621, -0.6224706135936574070, -0.1071654190663385853 ) ) ;
#6175=CARTESIAN_POINT ( 'NONE',  ( -0.5953962971613582233, -0.1370369651175855630, -0.2478037815953649248 ) ) ;
#6218=B_SPLINE_SURFACE_WITH_KNOTS ( 'NONE', 3, 3, ( 
 ( #1778, #15074, #10815, #4321, #4586 ),
 ( #13200, #14807, #10390, #19429, #5279 ),
 ( #22236, #2731, #26605, #2596, #379 ),
 ( #9092, #501, #15748, #20115, #9363 ) ),
 .UNSPECIFIED., .F., .F., .F.,
 ( 4, 4 ),
 ( 4, 1, 4 ),
 ( -0.5999999999999999778, 0.5999999999999999778 ),
 ( 1.887240170904915137, 3.034981381880270224, 4.565302996514080114 ),
 .UNSPECIFIED. ) ;
#6259=ADVANCED_FACE ( 'NONE', ( #5469 ), #16803, .F. ) ;
#6289=CARTESIAN_POINT ( 'NONE',  ( -0.4881018399981850719, -0.5317657191589535426, -0.05369922615894921064 ) ) ;
#6301=CARTESIAN_POINT ( 'NONE',  ( -0.5628483367911055746, -0.2097809568884774767, -0.2636329226663323144 ) ) ;
#6324=CARTESIAN_POINT ( 'NONE',  ( -0.7874015748031496509, 0.6226544199590670070, -0.5245967315940827103 ) ) ;
#6353=CARTESIAN_POINT ( 'NONE',  ( -0.3338887748335570560, 0.000000000000000000, -1.052618110236220428 ) ) ;
#6360=VERTEX_POINT ( 'NONE', #11965 ) ;
#6404=DIRECTION ( 'NONE',  ( 1.000000000000000000, 0.000000000000000000, 0.000000000000000000 ) ) ;
#6424=ORIENTED_EDGE ( 'NONE', *, *, #4318, .T. ) ;
#6425=CARTESIAN_POINT ( 'NONE',  ( -0.5355664161054535244, -0.4296723638627480413, 0.1626757613542834380 ) ) ;
#6434=FACE_OUTER_BOUND ( 'NONE', #12541, .T. ) ;
#6437=CARTESIAN_POINT ( 'NONE',  ( -0.6366897297587940097, -0.04473345904607178153, -0.2370953701923842472 ) ) ;
#6438=CARTESIAN_POINT ( 'NONE',  ( 0.1532705055535415473, -0.7132778159795964967, -0.1710911351452818752 ) ) ;
#6469=CARTESIAN_POINT ( 'NONE',  ( 0.3976891862754212137, 0.9951575781684135480, -0.5144425584461574941 ) ) ;
#6486=CIRCLE ( 'NONE', #26330, 1.288838582677166222 ) ;
#6493=EDGE_CURVE ( 'NONE', #27472, #5887, #19718, .T. ) ;
#6496=DIRECTION ( 'NONE',  ( 0.000000000000000000, 7.180547322999998243E-06, 0.9999999999742198442 ) ) ;
#6548=FACE_OUTER_BOUND ( 'NONE', #16522, .T. ) ;
#6553=EDGE_CURVE ( 'NONE', #26847, #15456, #2471, .T. ) ;
#6554=ORIENTED_EDGE ( 'NONE', *, *, #14242, .F. ) ;
#6561=VECTOR ( 'NONE', #26725, 39.37007874015748143 ) ;
#6565=CARTESIAN_POINT ( 'NONE',  ( -0.6562077975700453258, 2.612916929133858441E-14, 0.2362204724409449064 ) ) ;
#6573=CARTESIAN_POINT ( 'NONE',  ( -0.6587140840999922142, 0.007992779901115512273, 0.07874015870966120934 ) ) ;
#6591=VERTEX_POINT ( 'NONE', #1652 ) ;
#6621=VERTEX_POINT ( 'NONE', #18738 ) ;
#6625=CARTESIAN_POINT ( 'NONE',  ( 0.4563908000639795848, 0.8133290948875807613, -0.5151991767489622065 ) ) ;
#6627=CARTESIAN_POINT ( 'NONE',  ( 0.7266071376980735019, 0.7048822860824826009, 0.02652157274389425196 ) ) ;
#6641=CARTESIAN_POINT ( 'NONE',  ( -0.8725268807032540153, 0.000000000000000000, -1.052618110236220428 ) ) ;
#6646=CARTESIAN_POINT ( 'NONE',  ( 0.2249706821157846648, -0.8351807821610452987, -0.2761312587482271375 ) ) ;
#6657=VERTEX_POINT ( 'NONE', #9593 ) ;
#6714=CARTESIAN_POINT ( 'NONE',  ( -0.6912180915490531152, 0.1281909420063060967, 0.2299950541617507838 ) ) ;
#6720=CARTESIAN_POINT ( 'NONE',  ( 0.2249706821157846648, -0.7189271281445788198, -0.3842149643474468412 ) ) ;
#6761=CARTESIAN_POINT ( 'NONE',  ( 0.2083728861314909642, 0.3778799683988480762, -0.2992345713061846935 ) ) ;
#6764=CARTESIAN_POINT ( 'NONE',  ( 0.6343085930858298749, 0.8719994442144956004, -0.1034023825655943502 ) ) ;
#6824=CIRCLE ( 'NONE', #3636, 0.8163976377952757435 ) ;
#6825=CARTESIAN_POINT ( 'NONE',  ( -0.3338887748335582772, 0.000000000000000000, -1.052618110236220428 ) ) ;
#6850=CARTESIAN_POINT ( 'NONE',  ( -0.7795729917428700917, 0.3433105971656929545, -0.1409633029682732241 ) ) ;
#6861=DIRECTION ( 'NONE',  ( 1.000000000000000000, 0.000000000000000000, 0.000000000000000000 ) ) ;
#6898=CARTESIAN_POINT ( 'NONE',  ( 0.5985371529601012375, 0.9200311766420431470, -0.1500396732972504588 ) ) ;
#6914=DIRECTION ( 'NONE',  ( -1.000000000000000000, 0.000000000000000000, 0.000000000000000000 ) ) ;
#6937=CARTESIAN_POINT ( 'NONE',  ( 0.1120675189988344506, -0.4694218845611126678, -0.3846748511993472452 ) ) ;
#6951=ORIENTED_EDGE ( 'NONE', *, *, #7556, .F. ) ;
#6963=CARTESIAN_POINT ( 'NONE',  ( 0.4895462770358314786, 0.6604130065488427181, -0.5726600247966424639 ) ) ;
#6966=VECTOR ( 'NONE', #25462, 39.37007874015748143 ) ;
#6980=CARTESIAN_POINT ( 'NONE',  ( -0.6208708315385689236, -0.08043444190496674973, -0.2401670989486988372 ) ) ;
#6988=ORIENTED_EDGE ( 'NONE', *, *, #9138, .F. ) ;
#6991=CARTESIAN_POINT ( 'NONE',  ( -0.7121770198535963825, 0.1804934768145626256, 0.06452349730229350877 ) ) ;
#6994=PLANE ( 'NONE',  #16526 ) ;
#7030=CARTESIAN_POINT ( 'NONE',  ( 0.3843128886798082844, 0.1418101685954901714, -0.2362204724409449064 ) ) ;
#7083=EDGE_LOOP ( 'NONE', ( #25016, #2761, #459, #20214 ) ) ;
#7096=CARTESIAN_POINT ( 'NONE',  ( 0.7874015748031325534, 0.2480907742005069583, -0.2781032352068246172 ) ) ;
#7109=CARTESIAN_POINT ( 'NONE',  ( -0.6544535166833030937, -0.004815824195081693654, -0.07874015109845866611 ) ) ;
#7126=B_SPLINE_CURVE_WITH_KNOTS ( 'NONE', 3,
 ( #18186, #26826, #18618, #7476, #5508, #16104, #5360, #9733, #27123, #7769 ),
 .UNSPECIFIED., .F., .F.,
 ( 4, 2, 2, 2, 4 ),
 ( 0.000000000000000000, 0.2500000000000000000, 0.5000000000000000000, 0.7500000000000000000, 1.000000000000000000 ),
 .UNSPECIFIED. ) ;
#7138=ADVANCED_FACE ( 'NONE', ( #2362 ), #12508, .F. ) ;
#7140=AXIS2_PLACEMENT_3D ( 'NONE', #3235, #26845, #5384 ) ;
#7172=VECTOR ( 'NONE', #25980, 39.37007874015748143 ) ;
#7203=DIRECTION ( 'NONE',  ( 0.000000000000000000, -0.7626852297620279053, -0.6467698511084468693 ) ) ;
#7221=CARTESIAN_POINT ( 'NONE',  ( 0.7871730179869745880, 0.2557924603599555091, -0.2773276354974251734 ) ) ;
#7248=ADVANCED_FACE ( 'NONE', ( #4898 ), #23595, .T. ) ;
#7283=CARTESIAN_POINT ( 'NONE',  ( -0.7874015748031496509, 0.3943205132762559462, -0.07664873632799094894 ) ) ;
#7284=CARTESIAN_POINT ( 'NONE',  ( -0.3334645669291338987, 5.862181871850394349E-06, -1.869015748010449007 ) ) ;
#7295=CARTESIAN_POINT ( 'NONE',  ( -0.6562077975700453258, 2.612916929133858441E-14, 0.2362204724409449064 ) ) ;
#7296=CARTESIAN_POINT ( 'NONE',  ( -0.1786951194748074845, 0.7326758143698267611, -0.6802888381030000042 ) ) ;
#7305=VECTOR ( 'NONE', #20839, 39.37007874015748143 ) ;
#7347=CARTESIAN_POINT ( 'NONE',  ( -0.6513233937849554067, -0.01774504213867074409, 0.2362204724409449896 ) ) ;
#7364=EDGE_CURVE ( 'NONE', #27472, #550, #4616, .T. ) ;
#7365=CARTESIAN_POINT ( 'NONE',  ( 0.7873253891977465280, 0.2997731478012109485, -0.1260073171955472526 ) ) ;
#7390=CARTESIAN_POINT ( 'NONE',  ( -0.7874015748031496509, 0.4828108945773819105, 0.1423708153504031348 ) ) ;
#7419=CARTESIAN_POINT ( 'NONE',  ( -0.2070393714800602414, -0.1127906890684966662, 0.2362204724409449064 ) ) ;
#7426=CARTESIAN_POINT ( 'NONE',  ( -0.3528405259361242496, -0.7288848593461209058, -0.6846649188871202218 ) ) ;
#7431=CARTESIAN_POINT ( 'NONE',  ( -0.6996199877990079141, 0.1591959485999228652, 0.2265176967194976465 ) ) ;
#7443=ORIENTED_EDGE ( 'NONE', *, *, #4318, .F. ) ;
#7468=EDGE_CURVE ( 'NONE', #550, #6621, #16061, .T. ) ;
#7476=CARTESIAN_POINT ( 'NONE',  ( -0.4359497604187455022, 0.3683017918443335925, 0.1859854795144792461 ) ) ;
#7486=CARTESIAN_POINT ( 'NONE',  ( -0.6102864789886656149, -0.1643143352007618574, 0.2257035431949488136 ) ) ;
#7507=CARTESIAN_POINT ( 'NONE',  ( 0.6175000359513720394, 0.6841573636653760504, -0.3528259788121539398 ) ) ;
#7556=EDGE_CURVE ( 'NONE', #25001, #607, #1835, .T. ) ;
#7559=CARTESIAN_POINT ( 'NONE',  ( -0.4101012214746874163, -0.6863629600575589240, -0.3597087265456967997 ) ) ;
#7564=CARTESIAN_POINT ( 'NONE',  ( 0.7874015748031496509, 0.2962865104657910753, -0.1276405476038844355 ) ) ;
#7579=CARTESIAN_POINT ( 'NONE',  ( -0.03794311743615354227, 1.003836633634893838, -0.2033123174402287625 ) ) ;
#7583=CARTESIAN_POINT ( 'NONE',  ( 0.5979250048013408092, 0.9208089262530376740, -0.1508331457611719051 ) ) ;
#7595=CARTESIAN_POINT ( 'NONE',  ( -0.3361738726636556707, -1.237811886721866372, -0.6855454509606260238 ) ) ;
#7632=VERTEX_POINT ( 'NONE', #1501 ) ;
#7664=B_SPLINE_CURVE_WITH_KNOTS ( 'NONE', 3,
 ( #18134, #17995, #18283, #13930, #9532, #20707, #7426, #3174, #16468, #26634, #14364, #1087, #11664, #16053, #1354, #24511, #25081, #5161, #5747, #14074, #11150, #16196, #9827, #24796, #3311, #11953, #20572, #1226, #3893, #12367, #18851, #3598, #10383, #27351, #10523, #2051, #14937, #15071, #25787, #23118, #19002, #27636, #21412, #14803, #25218, #27775, #6301, #10662, #8004, #8281, #3748, #20843, #16900, #16605, #19285, #25510, #8553, #9311, #6175, #19142, #8143, #12227, #21129, #17173, #12649, #1493, #20986, #25648, #5889, #8416, #14515, #1632, #23546, #17037, #25363, #23409, #6025, #21276, #4041, #6437, #4180, #10237 ),
 .UNSPECIFIED., .F., .F.,
 ( 4, 2, 2, 2, 1, 1, 1, 1, 2, 2, 2, 2, 2, 1, 1, 1, 2, 2, 2, 2, 2, 1, 1, 2, 2, 2, 1, 1, 1, 2, 2, 2, 1, 1, 1, 1, 2, 2, 1, 1, 1, 1, 1, 2, 2, 2, 2, 1, 1, 1, 2, 2, 4 ),
 ( 0.000000000000000000, 0.1250000000000016098, 0.1875000000000022482, 0.2187500000000024702, 0.2343750000000026090, 0.2421875000000024980, 0.2460937500000025258, 0.2480468750000025258, 0.2490234375000025813, 0.2500000000000026090, 0.3750000000000124900, 0.4375000000000175415, 0.4687500000000200395, 0.4843750000000213163, 0.4921875000000219824, 0.4960937500000222600, 0.4980468750000223155, 0.5000000000000223155, 0.6250000000000152101, 0.6875000000000116573, 0.7187500000000097700, 0.7343750000000088818, 0.7421875000000084377, 0.7460937500000082157, 0.7500000000000078826, 0.7812500000000063283, 0.7968750000000054401, 0.8046875000000049960, 0.8085937500000048850, 0.8105468750000047740, 0.8125000000000046629, 0.8437500000000036637, 0.8593750000000031086, 0.8671875000000028866, 0.8710937500000026645, 0.8730468750000025535, 0.8740234375000025535, 0.8750000000000025535, 0.8906250000000015543, 0.8984375000000009992, 0.9023437500000007772, 0.9042968750000006661, 0.9052734375000005551, 0.9057617187500005551, 0.9062500000000005551, 0.9218749999999998890, 0.9296874999999995559, 0.9335937499999993339, 0.9355468749999994449, 0.9365234374999994449, 0.9370117187499994449, 0.9374999999999994449, 1.000000000000000000 ),
 .UNSPECIFIED. ) ;
#7668=DIRECTION ( 'NONE',  ( 0.000000000000000000, -7.180547322999999937E-06, -0.9999999999742198442 ) ) ;
#7679=ORIENTED_EDGE ( 'NONE', *, *, #21647, .F. ) ;
#7689=CARTESIAN_POINT ( 'NONE',  ( -0.2490711204941346568, 0.7655264129003995777, -0.7689379837741201484 ) ) ;
#7693=CARTESIAN_POINT ( 'NONE',  ( 0.5890517850735842442, -0.1846255037454771764, 0.07874015748031495954 ) ) ;
#7705=ADVANCED_FACE ( 'NONE', ( #23552 ), #10669, .F. ) ;
#7706=CARTESIAN_POINT ( 'NONE',  ( -0.6806799598997224088, 0.05663649493104071925, -0.2380830294301988226 ) ) ;
#7718=CARTESIAN_POINT ( 'NONE',  ( -0.3338887748335582772, -5.862181872755905604E-06, -1.869015748010449007 ) ) ;
#7742=DIRECTION ( 'NONE',  ( -1.000000000000000000, 0.000000000000000000, 0.000000000000000000 ) ) ;
#7743=ORIENTED_EDGE ( 'NONE', *, *, #16614, .F. ) ;
#7769=CARTESIAN_POINT ( 'NONE',  ( -0.7874015748031496509, 0.9829781505553011334, -0.2190361720152886049 ) ) ;
#7797=ADVANCED_FACE ( 'NONE', ( #26066 ), #6218, .F. ) ;
#7819=CARTESIAN_POINT ( 'NONE',  ( 0.3976891862754212137, 0.8566358266442657410, -0.5893543329197449276 ) ) ;
#7820=EDGE_CURVE ( 'NONE', #22680, #24641, #6824, .T. ) ;
#7838=AXIS2_PLACEMENT_3D ( 'NONE', #6353, #16809, #25565 ) ;
#7848=CARTESIAN_POINT ( 'NONE',  ( -0.3376790527244098450, -1.225034693736185121, -0.6364355922310138691 ) ) ;
#7853=CIRCLE ( 'NONE', #24093, 0.8163976377952757435 ) ;
#7858=CARTESIAN_POINT ( 'NONE',  ( 0.1120675189988346587, -0.5599717622282432972, -0.2558308786799980417 ) ) ;
#7881=B_SPLINE_CURVE_WITH_KNOTS ( 'NONE', 3,
 ( #17517, #4251, #8483, #1984, #12856, #26135 ),
 .UNSPECIFIED., .F., .F.,
 ( 4, 2, 4 ),
 ( -1.199999999999999956, -0.5999999999999999778, 0.000000000000000000 ),
 .UNSPECIFIED. ) ;
#7890=ORIENTED_EDGE ( 'NONE', *, *, #23474, .T. ) ;
#7916=CARTESIAN_POINT ( 'NONE',  ( -0.5385832331986013521, -0.4187149276795443242, 0.1663235595950885437 ) ) ;
#7923=DIRECTION ( 'NONE',  ( 1.000000000000000000, 0.000000000000000000, 0.000000000000000000 ) ) ;
#7933=DIRECTION ( 'NONE',  ( -1.000000000000000000, 0.000000000000000000, 0.000000000000000000 ) ) ;
#7953=ADVANCED_FACE ( 'NONE', ( #3717 ), #20838, .T. ) ;
#7974=CYLINDRICAL_SURFACE ( 'NONE', #16940, 0.8163976377952756325 ) ;
#7988=CARTESIAN_POINT ( 'NONE',  ( -0.5172021183779732523, -0.4971257496141905929, 0.1366764242586682998 ) ) ;
#7999=CARTESIAN_POINT ( 'NONE',  ( -0.2070393714800602414, -0.07144576004975727868, -0.2362204724409449064 ) ) ;
#8004=CARTESIAN_POINT ( 'NONE',  ( -0.5638480983043335781, -0.2075177900316160229, -0.2630347114838766931 ) ) ;
#8015=CARTESIAN_POINT ( 'NONE',  ( -0.3334645669291338987, 0.8103892183150610551, -0.9220603341868013336 ) ) ;
#8061=CARTESIAN_POINT ( 'NONE',  ( -0.6035792859986336412, -0.1877841116824367773, 0.2224687983481839493 ) ) ;
#8081=CARTESIAN_POINT ( 'NONE',  ( 0.4895462770358314786, 0.6565912641725563104, -0.5754374930411751965 ) ) ;
#8103=DIRECTION ( 'NONE',  ( 0.000000000000000000, 0.9999999999742198442, -7.180547322999998243E-06 ) ) ;
#8106=EDGE_LOOP ( 'NONE', ( #23699, #4496, #15215, #3011 ) ) ;
#8113=( NAMED_UNIT ( * ) PLANE_ANGLE_UNIT ( ) SI_UNIT ( $, .RADIAN. ) ) ;
#8125=CARTESIAN_POINT ( 'NONE',  ( -0.5743180011325290657, -0.2548351232479605932, 0.04982753927068897526 ) ) ;
#8143=CARTESIAN_POINT ( 'NONE',  ( -0.6020026763137992232, -0.1224252381418852453, -0.2454157907868443067 ) ) ;
#8156=DIRECTION ( 'NONE',  ( 0.000000000000000000, -0.9999999999742198442, -7.180547322999998243E-06 ) ) ;
#8205=( NAMED_UNIT ( * ) PLANE_ANGLE_UNIT ( ) SI_UNIT ( $, .RADIAN. ) ) ;
#8258=CARTESIAN_POINT ( 'NONE',  ( -0.3334645669291338987, 1.279353152430305007, -0.8465078874097147210 ) ) ;
#8262=ORIENTED_EDGE ( 'NONE', *, *, #20508, .F. ) ;
#8263=CARTESIAN_POINT ( 'NONE',  ( -0.6002615430280354714, -0.1750105204655757751, 0.06519039343118070151 ) ) ;
#8281=CARTESIAN_POINT ( 'NONE',  ( -0.5688514329716306550, -0.1961983850004131169, -0.2600699532609946907 ) ) ;
#8307=CARTESIAN_POINT ( 'NONE',  ( -0.5677441908128973980, 0.3966471237414492257, -0.3366160073295133004 ) ) ;
#8336=CARTESIAN_POINT ( 'NONE',  ( 0.7874015748031496509, 0.000000000000000000, 0.2362204724409449619 ) ) ;
#8339=CARTESIAN_POINT ( 'NONE',  ( -0.4325335578080637955, -0.8196558064895489437, -0.05799776393766782612 ) ) ;
#8378=VERTEX_POINT ( 'NONE', #12623 ) ;
#8405=CARTESIAN_POINT ( 'NONE',  ( -0.6068752646683485130, -0.1547367907410470145, 0.06814449279195373965 ) ) ;
#8411=CARTESIAN_POINT ( 'NONE',  ( -0.2602238532265429005, 0.000000000000000000, 0.2362204724409449064 ) ) ;
#8416=CARTESIAN_POINT ( 'NONE',  ( -0.6149721272769592684, -0.09366413789291816450, -0.2415914643636047077 ) ) ;
#8456=CARTESIAN_POINT ( 'NONE',  ( 0.4563908000639795848, 1.076366897322332816, -0.3413933471944003428 ) ) ;
#8483=CARTESIAN_POINT ( 'NONE',  ( -0.6562077975700374433, -2.731848031496062854E-17, -0.07874015748031495954 ) ) ;
#8490=LINE ( 'NONE', #14338, #25043 ) ;
#8512=DIRECTION ( 'NONE',  ( 0.000000000000000000, 0.7626852297620280163, 0.6467698511084468693 ) ) ;
#8536=EDGE_CURVE ( 'NONE', #4501, #22748, #14225, .T. ) ;
#8540=CARTESIAN_POINT ( 'NONE',  ( -0.5546128944410685380, -0.2725325685736035286, -0.1175119830017629929 ) ) ;
#8553=CARTESIAN_POINT ( 'NONE',  ( -0.5948382950512706158, -0.1382708294208072619, -0.2480148272232753359 ) ) ;
#8556=CARTESIAN_POINT ( 'NONE',  ( 0.1532705055535415473, -0.5147072688414000563, -0.4165008336377047371 ) ) ;
#8559=EDGE_CURVE ( 'NONE', #24641, #17699, #2050, .T. ) ;
#8574=CARTESIAN_POINT ( 'NONE',  ( 0.7874015748031496509, -0.3839064563524838825, -0.3321176343386787466 ) ) ;
#8585=CARTESIAN_POINT ( 'NONE',  ( 0.3339160553493882300, 1.214868409966151530, -0.6104964979807637748 ) ) ;
#8599=VECTOR ( 'NONE', #16469, 39.37007874015748854 ) ;
#8612=ORIENTED_EDGE ( 'NONE', *, *, #25937, .F. ) ;
#8649=ADVANCED_FACE ( 'NONE', ( #6548 ), #12040, .F. ) ;
#8674=CARTESIAN_POINT ( 'NONE',  ( -0.6562077975700453258, 2.293650393700787223E-14, 0.07874015748031495954 ) ) ;
#8686=CARTESIAN_POINT ( 'NONE',  ( -0.7635713814939685262, 0.3473852540523503785, 0.02512505594370720644 ) ) ;
#8688=VECTOR ( 'NONE', #2672, 39.37007874015748854 ) ;
#8692=CARTESIAN_POINT ( 'NONE',  ( 0.3102399269716953345, -1.013856135328759844, -0.5158482079756747662 ) ) ;
#8695=DIRECTION ( 'NONE',  ( 1.000000000000000000, 0.000000000000000000, 0.000000000000000000 ) ) ;
#8735=CARTESIAN_POINT ( 'NONE',  ( 0.7772278266253901391, 0.5213247747914033781, 0.1262149107176392671 ) ) ;
#8737=AXIS2_PLACEMENT_3D ( 'NONE', #5042, #22143, #22279 ) ;
#8744=CARTESIAN_POINT ( 'NONE',  ( -0.3700489919980719522, -1.073999312313020926, -0.3399043508710541950 ) ) ;
#8748=AXIS2_PLACEMENT_3D ( 'NONE', #2953, #11584, #13700 ) ;
#8752=FACE_OUTER_BOUND ( 'NONE', #21072, .T. ) ;
#8765=FACE_OUTER_BOUND ( 'NONE', #17023, .T. ) ;
#8770=DIRECTION ( 'NONE',  ( 0.000000000000000000, 7.180547322999999937E-06, -0.9999999999742198442 ) ) ;
#8771=CARTESIAN_POINT ( 'NONE',  ( -0.3334645669291338987, 9.254566433503937147E-06, -2.341456692880161228 ) ) ;
#8773=ADVANCED_FACE ( 'NONE', ( #20644 ), #3830, .T. ) ;
#8784=LINE ( 'NONE', #15318, #23662 ) ;
#8812=CARTESIAN_POINT ( 'NONE',  ( -0.6505662911506299162, -0.01547120374406815019, -0.07881933527123072269 ) ) ;
#8819=AXIS2_PLACEMENT_3D ( 'NONE', #13261, #6914, #4634 ) ;
#8821=CARTESIAN_POINT ( 'NONE',  ( -0.7795729917428700917, 0.4543402377591519992, 0.1538738033641767755 ) ) ;
#8824=DIRECTION ( 'NONE',  ( 0.000000000000000000, 0.9850313626640179177, -0.1723752144836030176 ) ) ;
#8825=CARTESIAN_POINT ( 'NONE',  ( 0.3334645669291338987, -1.269546425348450747, -0.8304542831125020230 ) ) ;
#8865=CARTESIAN_POINT ( 'NONE',  ( 0.3976891862754212137, 1.133679329692560911, -0.4395307839725701160 ) ) ;
#8866=CARTESIAN_POINT ( 'NONE',  ( 0.6936167303942817330, 0.7750952645509693317, -0.02289373067002851980 ) ) ;
#8875=CARTESIAN_POINT ( 'NONE',  ( -0.3724354128627712091, -1.063775794758070603, -0.3247274185435837235 ) ) ;
#8878=DIRECTION ( 'NONE',  ( 0.000000000000000000, 0.000000000000000000, 1.000000000000000000 ) ) ;
#8891=CARTESIAN_POINT ( 'NONE',  ( 0.7871730179869745880, 0.4038169352867496120, 0.1713250154738354125 ) ) ;
#8926=CARTESIAN_POINT ( 'NONE',  ( -0.1981752911889803348, -0.08335338672471442889, -0.2362204724409444623 ) ) ;
#8930=CARTESIAN_POINT ( 'NONE',  ( 0.3334645669291338987, -1.269546425348450747, -0.8304542831125020230 ) ) ;
#8942=CARTESIAN_POINT ( 'NONE',  ( -0.6112138326843681302, -0.1413929495357376109, 0.06990500580186909119 ) ) ;
#8986=CARTESIAN_POINT ( 'NONE',  ( -0.3334645669291338987, 0.000000000000000000, -1.052618110236220428 ) ) ;
#9063=CARTESIAN_POINT ( 'NONE',  ( 0.4895462770358314786, 0.9151958316345965017, -0.3874954751611386361 ) ) ;
#9087=CARTESIAN_POINT ( 'NONE',  ( -0.6562077975700097987, -9.864972440944882481E-14, 0.2362204724409449064 ) ) ;
#9092=CARTESIAN_POINT ( 'NONE',  ( -0.2602238532265429005, 0.000000000000000000, 0.2362204724409449064 ) ) ;
#9128=CARTESIAN_POINT ( 'NONE',  ( 0.4898768902087983768, -3.758337795275590876E-16, 0.07874015748031495954 ) ) ;
#9130=CARTESIAN_POINT ( 'NONE',  ( 0.7611552401864779549, 0.5997378224220212273, 0.08818015398314092701 ) ) ;
#9134=AXIS2_PLACEMENT_3D ( 'NONE', #23819, #8695, #19848 ) ;
#9138=EDGE_CURVE ( 'NONE', #26345, #4501, #17651, .T. ) ;
#9183=CARTESIAN_POINT ( 'NONE',  ( 0.3334645669291338987, -1.269546425348450747, -0.8304542831125020230 ) ) ;
#9192=CARTESIAN_POINT ( 'NONE',  ( 0.7871730179869745880, 0.2552990454435328793, -0.2788231443339960758 ) ) ;
#9206=CARTESIAN_POINT ( 'NONE',  ( -0.6434710025615986151, -0.04612040742723353542, 0.2355049364185476390 ) ) ;
#9262=CARTESIAN_POINT ( 'NONE',  ( 0.6667153566691432776, 0.8231464062114414171, -0.06035729286437391955 ) ) ;
#9311=CARTESIAN_POINT ( 'NONE',  ( -0.5951974299326810991, -0.1374766578026193065, -0.2478787525163752559 ) ) ;
#9313=ORIENTED_EDGE ( 'NONE', *, *, #4049, .T. ) ;
#9325=CARTESIAN_POINT ( 'NONE',  ( 0.7845931698711713365, 0.3305999548149256562, -0.3053253099640526602 ) ) ;
#9357=DIRECTION ( 'NONE',  ( 0.000000000000000000, -0.9850313626640178066, 0.1723752144836030453 ) ) ;
#9363=CARTESIAN_POINT ( 'NONE',  ( -0.7874015748031496509, 0.9829781505553011334, -0.2190361720152889935 ) ) ;
#9380=EDGE_CURVE ( 'NONE', #6360, #6657, #26288, .T. ) ;
#9400=CIRCLE ( 'NONE', #2203, 0.8163976377952758545 ) ;
#9401=CARTESIAN_POINT ( 'NONE',  ( 0.5797993700277297435, 0.9434079930944230252, -0.1743634797089741728 ) ) ;
#9407=FACE_OUTER_BOUND ( 'NONE', #19092, .T. ) ;
#9467=CARTESIAN_POINT ( 'NONE',  ( 0.6175000359513720394, 0.5702072523746822830, -0.4693776984553832410 ) ) ;
#9479=CARTESIAN_POINT ( 'NONE',  ( -0.8725268807032540153, 0.000000000000000000, -0.2362204724409448231 ) ) ;
#9519=CARTESIAN_POINT ( 'NONE',  ( -0.4101012214746874163, -0.9083388034714960924, -0.1356156739343915285 ) ) ;
#9528=CARTESIAN_POINT ( 'NONE',  ( -0.2070393714800602414, -0.09900904606225019444, 0.07874015748031495954 ) ) ;
#9532=CARTESIAN_POINT ( 'NONE',  ( -0.3458583018457046521, -0.7501511824813903440, -0.7295201136257942753 ) ) ;
#9552=CARTESIAN_POINT ( 'NONE',  ( 0.4898768902087983768, 0.000000000000000000, -0.2362204724409449064 ) ) ;
#9568=ORIENTED_EDGE ( 'NONE', *, *, #20277, .F. ) ;
#9572=AXIS2_PLACEMENT_3D ( 'NONE', #14638, #12763, #17010 ) ;
#9589=CARTESIAN_POINT ( 'NONE',  ( -0.6142148233928379497, -0.1505053300589599685, 0.2274168496461167199 ) ) ;
#9593=CARTESIAN_POINT ( 'NONE',  ( 0.7874015748031496509, -3.035194737559056185E-06, -1.475314960619023674 ) ) ;
#9610=CARTESIAN_POINT ( 'NONE',  ( 0.7845931698711713365, 0.3318803385907665437, -0.3024313949403425461 ) ) ;
#9611=B_SPLINE_CURVE_WITH_KNOTS ( 'NONE', 3,
 ( #9855, #12117, #18747, #24967 ),
 .UNSPECIFIED., .F., .F.,
 ( 4, 4 ),
 ( 0.000000000000000000, 1.000000000000000000 ),
 .UNSPECIFIED. ) ;
#9633=CARTESIAN_POINT ( 'NONE',  ( 0.4245040230929275626, 1.106753849019775471, -0.3897420188601015689 ) ) ;
#9647=B_SPLINE_CURVE_WITH_KNOTS ( 'NONE', 3,
 ( #27372, #8926, #15036, #10917, #4286, #2690 ),
 .UNSPECIFIED., .F., .F.,
 ( 4, 2, 4 ),
 ( 0.000000000000000000, 0.5000000000000000000, 1.000000000000000000 ),
 .UNSPECIFIED. ) ;
#9655=EDGE_CURVE ( 'NONE', #21760, #13891, #21780, .T. ) ;
#9671=CARTESIAN_POINT ( 'NONE',  ( -0.3681444341728476455, -0.6850021075794429093, -0.6051803271985433108 ) ) ;
#9680=CARTESIAN_POINT ( 'NONE',  ( -0.2602238532265429005, 0.000000000000000000, -0.2362204724409449064 ) ) ;
#9694=CARTESIAN_POINT ( 'NONE',  ( 0.4898768902087983768, -4.281484251968504304E-16, 0.2362204724409449064 ) ) ;
#9697=CARTESIAN_POINT ( 'NONE',  ( 0.5485639935000311551, 0.9796862869722393619, -0.2151333194223323253 ) ) ;
#9733=CARTESIAN_POINT ( 'NONE',  ( -0.6995386212070490162, 0.8547296533447173994, -0.08348329912257269891 ) ) ;
#9736=CARTESIAN_POINT ( 'NONE',  ( -0.7874015748031496509, 0.9829781505553011334, -0.2190361720152889935 ) ) ;
#9815=CARTESIAN_POINT ( 'NONE',  ( -0.3376790527244098450, -0.7759819139694350554, -0.7889928361655353939 ) ) ;
#9827=CARTESIAN_POINT ( 'NONE',  ( -0.4251109113156978370, -0.5377216242369684540, -0.4382667117914157418 ) ) ;
#9831=CARTESIAN_POINT ( 'NONE',  ( -0.7635713814939685262, 0.3957398197978322374, 0.1751423728567907401 ) ) ;
#9836=AXIS2_PLACEMENT_3D ( 'NONE', #24389, #16065, #19504 ) ;
#9843=AXIS2_PLACEMENT_3D ( 'NONE', #9183, #11734, #591 ) ;
#9855=CARTESIAN_POINT ( 'NONE',  ( -0.3334645669291338987, 0.8151331854455394765, -1.007197927683596506 ) ) ;
#9856=ORIENTED_EDGE ( 'NONE', *, *, #1800, .T. ) ;
#9893=VECTOR ( 'NONE', #15625, 39.37007874015748143 ) ;
#9944=PRODUCT_DEFINITION_CONTEXT ( 'detailed design', #21908, 'design' ) ;
#9952=CARTESIAN_POINT ( 'NONE',  ( -0.4473595089310440920, -0.6685828274113149172, -0.1391927031366795575 ) ) ;
#9965=ORIENTED_EDGE ( 'NONE', *, *, #10875, .T. ) ;
#9977=CARTESIAN_POINT ( 'NONE',  ( -0.2490711204941342405, 1.208528701367826752, -0.6047752023237676910 ) ) ;
#10002=CARTESIAN_POINT ( 'NONE',  ( 0.3769281224616271575, 0.7313191576793038884, -0.6886840467356212248 ) ) ;
#10024=CARTESIAN_POINT ( 'NONE',  ( -0.6081663209497759626, -0.1717464423132456786, 0.2247343301158596096 ) ) ;
#10029=AXIS2_PLACEMENT_3D ( 'NONE', #22224, #19969, #17577 ) ;
#10039=CARTESIAN_POINT ( 'NONE',  ( 0.7874015748031496509, -5.862181872755905604E-06, -1.869015748010449007 ) ) ;
#10063=ORIENTED_EDGE ( 'NONE', *, *, #1754, .T. ) ;
#10079=VECTOR ( 'NONE', #2238, 39.37007874015748143 ) ;
#10082=ORIENTED_EDGE ( 'NONE', *, *, #21507, .F. ) ;
#10131=ORIENTED_EDGE ( 'NONE', *, *, #22612, .F. ) ;
#10157=EDGE_CURVE ( 'NONE', #24360, #22680, #18939, .T. ) ;
#10161=VECTOR ( 'NONE', #14029, 39.37007874015748854 ) ;
#10164=EDGE_CURVE ( 'NONE', #5599, #607, #5966, .T. ) ;
#10222=CARTESIAN_POINT ( 'NONE',  ( -0.5172021183779732523, -0.4363830659385236621, -0.008640819949054292723 ) ) ;
#10237=CARTESIAN_POINT ( 'NONE',  ( -0.6562077975700374433, -1.365924015748031427E-17, -0.2362204724409449064 ) ) ;
#10251=CARTESIAN_POINT ( 'NONE',  ( 0.7845931698711713365, 0.3318803385907665437, -0.3024313949403425461 ) ) ;
#10292=CARTESIAN_POINT ( 'NONE',  ( -0.5941926817969179764, -0.2205403317192303758, 0.2172113851610799617 ) ) ;
#10311=DIMENSIONAL_EXPONENTS ( 1.000000000000000000, 0.000000000000000000, 0.000000000000000000, 0.000000000000000000, 0.000000000000000000, 0.000000000000000000, 0.000000000000000000 ) ;
#10368=CARTESIAN_POINT ( 'NONE',  ( -0.5743180011325290657, -0.2193631536940708893, -0.1036282081129438898 ) ) ;
#10379=ORIENTED_EDGE ( 'NONE', *, *, #21049, .T. ) ;
#10383=CARTESIAN_POINT ( 'NONE',  ( -0.5098050478186216816, -0.3322734260891199165, -0.3067987715593742948 ) ) ;
#10390=CARTESIAN_POINT ( 'NONE',  ( -0.5112608635011182123, 0.4023796438212055016, -0.1315133041178671303 ) ) ;
#10398=B_SPLINE_CURVE_WITH_KNOTS ( 'NONE', 3,
 ( #11987, #3786, #12406, #12259, #10002, #14405 ),
 .UNSPECIFIED., .F., .F.,
 ( 4, 2, 4 ),
 ( 0.000000000000000000, 0.5000000000000000000, 1.000000000000000000 ),
 .UNSPECIFIED. ) ;
#10426=EDGE_CURVE ( 'NONE', #24641, #16499, #10398, .T. ) ;
#10462=DIRECTION ( 'NONE',  ( -1.000000000000000000, 0.000000000000000000, 0.000000000000000000 ) ) ;
#10463=ORIENTED_EDGE ( 'NONE', *, *, #7468, .T. ) ;
#10473=B_SPLINE_SURFACE_WITH_KNOTS ( 'NONE', 3, 3, ( 
 ( #20411, #24923, #14213, #27337 ),
 ( #24636, #22392, #15893, #3161 ),
 ( #9815, #22819, #3438, #7848 ),
 ( #20694, #24496, #5448, #3014 ),
 ( #9671, #13920, #18414, #11652 ),
 ( #22535, #18116, #20271, #16040 ),
 ( #12075, #7559, #18554, #9519 ),
 ( #5295, #16184, #22673, #3300 ),
 ( #1210, #1344, #9952, #27199 ),
 ( #16457, #25207, #6164, #18838 ),
 ( #19271, #25774, #21261, #23532 ),
 ( #14647, #1898, #6289, #4165 ),
 ( #19414, #12772, #4303, #25500 ),
 ( #18326, #3881, #6010, #10505 ),
 ( #21398, #23250, #10222, #7988 ),
 ( #12910, #4026, #10796, #23394 ),
 ( #14922, #19128, #12636, #6425 ),
 ( #10651, #27480, #16734, #2039 ),
 ( #1756, #8540, #21115, #23669 ),
 ( #15057, #21535, #17158, #2183 ),
 ( #16594, #10368, #8125, #5873 ),
 ( #25347, #14501, #27762, #23105 ),
 ( #3733, #12356, #18989, #20975 ),
 ( #1618, #27622, #8263, #12500 ),
 ( #16887, #14791, #8405, #17024 ),
 ( #25636, #4701, #8942, #4979 ),
 ( #13595, #10933, #15732, #22217 ),
 ( #6980, #13456, #15467, #17828 ),
 ( #21677, #24204, #2711, #26445 ),
 ( #19824, #2578, #26184, #19554 ),
 ( #236, #485, #17292, #2844 ),
 ( #4569, #24066, #26044, #9206 ),
 ( #13328, #8812, #104, #21811 ),
 ( #11075, #7109, #25914, #24335 ),
 ( #11482, #15187, #8674, #6565 ) ),
 .UNSPECIFIED., .F., .F., .F.,
 ( 4, 1, 1, 1, 1, 1, 1, 1, 1, 1, 1, 1, 1, 1, 1, 1, 1, 1, 1, 1, 1, 1, 1, 1, 1, 1, 1, 1, 1, 1, 1, 1, 4 ),
 ( 4, 4 ),
 ( 1.918259199999999943E-08, 0.04098565352343399443, 0.08197128786427600178, 0.1024641050346969950, 0.1434497393755389816, 0.1639425565459600165, 0.1946817823015919990, 0.2049281908868030022, 0.2254210080572240094, 0.2356674166424339856, 0.2510370295202500324, 0.2561602338128550205, 0.2664066423980660514, 0.2715298466906710395, 0.2817762552758819594, 0.2868994595684870030, 0.2971458681536969793, 0.3022690724463030221, 0.3125154810315129983, 0.3176386853241179864, 0.3278850939093290173, 0.3330082982019340054, 0.3406931046408420150, 0.3432547067871450364, 0.3483779110797499690, 0.3509395132260529904, 0.3560627175186579785, 0.3586243196649609999, 0.3637475239575660435, 0.3663091261038680102, 0.3739939325427759642, 0.3791171368353820070, 0.3833360769390560252 ),
 ( -0.5999999999999999778, 0.5999999999999999778 ),
 .UNSPECIFIED. ) ;
#10478=ORIENTED_EDGE ( 'NONE', *, *, #24264, .T. ) ;
#10505=CARTESIAN_POINT ( 'NONE',  ( -0.5072939182192724994, -0.5338842954723621581, 0.1206349394395838659 ) ) ;
#10523=CARTESIAN_POINT ( 'NONE',  ( -0.5218358954157312768, -0.3040829563514129141, -0.2949399236599603569 ) ) ;
#10526=ADVANCED_FACE ( 'NONE', ( #25822 ), #19046, .T. ) ;
#10529=CARTESIAN_POINT ( 'NONE',  ( 0.3334645669291338987, -1.243457723967850148, -0.6813714283177954023 ) ) ;
#10562=ORIENTED_EDGE ( 'NONE', *, *, #15166, .T. ) ;
#10571=EDGE_CURVE ( 'NONE', #15240, #10641, #26266, .T. ) ;
#10576=CARTESIAN_POINT ( 'NONE',  ( -0.5833027994817057138, -0.2586580032347411962, 0.2101318059641304747 ) ) ;
#10600=DIRECTION ( 'NONE',  ( 0.000000000000000000, 0.4702444477782121712, -0.8825362085114493160 ) ) ;
#10641=VERTEX_POINT ( 'NONE', #7284 ) ;
#10651=CARTESIAN_POINT ( 'NONE',  ( -0.5439522672647024715, -0.2528481198474323288, -0.2762448575629318781 ) ) ;
#10662=CARTESIAN_POINT ( 'NONE',  ( -0.5634947805916841190, -0.2083173938535096414, -0.2632452328862202595 ) ) ;
#10667=CARTESIAN_POINT ( 'NONE',  ( 0.3102399269716953345, -0.8727316232512619676, -0.5905643219437008984 ) ) ;
#10669=PLANE ( 'NONE',  #2739 ) ;
#10674=B_SPLINE_CURVE_WITH_KNOTS ( 'NONE', 3,
 ( #717, #7347, #24705, #24570, #20626, #17910, #18484, #15825, #26687, #5222, #999, #9589, #1142, #18197, #7486, #16385, #18339, #14134, #6087, #3509, #10024, #16517, #1831, #12139, #8061, #19055, #16813, #25568, #18773, #16672, #17086, #27554, #1404, #25281, #18625, #5657, #14725, #12700, #10292, #14577, #10576, #23176, #23328, #25139, #14282, #27829, #5801, #21041, #27262, #3954, #18913, #22892, #14851, #7916, #14426, #16952, #19200, #3655, #23467, #5942, #20905, #21333, #1688, #23032, #1967, #12430, #21189, #3811, #27688, #4094, #12283, #8339, #1549, #23732, #4236, #171, #8875, #8744, #13387, #42, #22015, #17364, #26113, #21743, #11276, #12975, #11002, #1108, #7595, #3049, #5333 ),
 .UNSPECIFIED., .F., .F.,
 ( 4, 2, 1, 1, 2, 2, 1, 1, 1, 1, 1, 1, 2, 2, 2, 2, 1, 1, 1, 2, 2, 2, 1, 1, 1, 2, 2, 2, 1, 1, 1, 1, 2, 2, 2, 1, 1, 1, 2, 2, 2, 2, 2, 1, 1, 1, 1, 2, 2, 2, 2, 2, 1, 1, 1, 1, 2, 2, 2, 4 ),
 ( 0.000000000000000000, 0.03125000000001444678, 0.04687500000002166323, 0.05468750000002530615, 0.05859375000002713801, 0.06250000000002896294, 0.07812500000003637368, 0.08593750000004005130, 0.08984375000004191092, 0.09179687500004279910, 0.09277343750004320155, 0.09326171875004343748, 0.09350585937504350686, 0.09375000000004357625, 0.1015625000000450612, 0.1054687500000458245, 0.1074218750000461992, 0.1083984375000463934, 0.1088867187500464906, 0.1091308593750465322, 0.1093750000000465739, 0.1171875000000476841, 0.1210937500000482531, 0.1230468750000485167, 0.1240234375000486139, 0.1245117187500486694, 0.1250000000000487110, 0.1562500000000492661, 0.1718750000000495992, 0.1796875000000497935, 0.1835937500000499600, 0.1855468750000500711, 0.1865234375000500988, 0.1875000000000500988, 0.2187500000000488221, 0.2343750000000482114, 0.2421875000000479061, 0.2460937500000477673, 0.2480468750000476841, 0.2500000000000476286, 0.3750000000000428546, 0.4375000000000404676, 0.4687500000000393019, 0.4843750000000386913, 0.4921875000000383582, 0.4960937500000381917, 0.4980468750000381362, 0.4990234375000380251, 0.5000000000000378586, 0.6250000000000266454, 0.6875000000000210942, 0.7187500000000183187, 0.7343750000000169864, 0.7421875000000162093, 0.7460937500000158762, 0.7480468750000156541, 0.7490234375000155431, 0.7500000000000154321, 0.8750000000000076605, 1.000000000000000000 ),
 .UNSPECIFIED. ) ;
#10691=CARTESIAN_POINT ( 'NONE',  ( 0.7874015748031496509, 0.3931603432736094361, 0.1747896609116821598 ) ) ;
#10724=EDGE_CURVE ( 'NONE', #26289, #25001, #14359, .T. ) ;
#10756=ADVANCED_FACE ( 'NONE', ( #22830 ), #27165, .F. ) ;
#10767=B_SPLINE_CURVE_WITH_KNOTS ( 'NONE', 3,
 ( #16367, #24970, #3785, #25116 ),
 .UNSPECIFIED., .F., .F.,
 ( 4, 4 ),
 ( 0.000000000000000000, 0.0002837997277716974506 ),
 .UNSPECIFIED. ) ;
#10772=FACE_OUTER_BOUND ( 'NONE', #24118, .T. ) ;
#10776=ORIENTED_EDGE ( 'NONE', *, *, #13942, .T. ) ;
#10781=LINE ( 'NONE', #17559, #21139 ) ;
#10796=CARTESIAN_POINT ( 'NONE',  ( -0.5252801253069795395, -0.4102412259628235858, 0.001906318767970118216 ) ) ;
#10807=CARTESIAN_POINT ( 'NONE',  ( -0.7432982829791772161, 0.3208553412839740826, 0.1963361843227200976 ) ) ;
#10808=ORIENTED_EDGE ( 'NONE', *, *, #578, .T. ) ;
#10812=CARTESIAN_POINT ( 'NONE',  ( 0.3334645669291338987, -1.269546425348450747, -0.8304542831125020230 ) ) ;
#10815=CARTESIAN_POINT ( 'NONE',  ( -0.5112608635011182123, 0.3373130994319499809, -0.2804599709653767814 ) ) ;
#10842=CARTESIAN_POINT ( 'NONE',  ( 0.3339160553493882300, 1.090203750159222551, -0.7502486126520099274 ) ) ;
#10875=EDGE_CURVE ( 'NONE', #4501, #26847, #23528, .T. ) ;
#10878=DIMENSIONAL_EXPONENTS ( 1.000000000000000000, 0.000000000000000000, 0.000000000000000000, 0.000000000000000000, 0.000000000000000000, 0.000000000000000000, 0.000000000000000000 ) ;
#10908=AXIS2_PLACEMENT_3D ( 'NONE', #14298, #3678, #3531 ) ;
#10917=CARTESIAN_POINT ( 'NONE',  ( -0.01202960507629146671, -0.3256422846268542948, -0.2993518939891427477 ) ) ;
#10933=CARTESIAN_POINT ( 'NONE',  ( -0.6165893942483189338, -0.1074060693884885814, -0.08465106059891655543 ) ) ;
#10942=ADVANCED_FACE ( 'NONE', ( #22087 ), #4578, .F. ) ;
#10945=CARTESIAN_POINT ( 'NONE',  ( -0.6912180915490531152, 0.08120084520073209133, -0.2401638807511342344 ) ) ;
#10952=CARTESIAN_POINT ( 'NONE',  ( 0.1120675189988346587, -0.6505216398953739265, -0.1269869061606480332 ) ) ;
#10961=ORIENTED_EDGE ( 'NONE', *, *, #20824, .T. ) ;
#10962=LINE ( 'NONE', #12802, #1014 ) ;
#10996=CARTESIAN_POINT ( 'NONE',  ( 0.4245040230929275626, 1.106753849019775471, -0.3897420188601015689 ) ) ;
#11002=CARTESIAN_POINT ( 'NONE',  ( -0.3521695574743459733, -1.152827357733649638, -0.4707598252271103512 ) ) ;
#11027=CARTESIAN_POINT ( 'NONE',  ( -0.6562077975700453258, 2.612916929133858441E-14, 0.2362204724409449064 ) ) ;
#11049=CARTESIAN_POINT ( 'NONE',  ( -0.7874015748031496509, 3.035194737559056185E-06, -1.475314960619023674 ) ) ;
#11050=DIRECTION ( 'NONE',  ( -1.000000000000000000, 0.000000000000000000, 0.000000000000000000 ) ) ;
#11071=EDGE_CURVE ( 'NONE', #26673, #16499, #5289, .T. ) ;
#11075=CARTESIAN_POINT ( 'NONE',  ( -0.6544535166833030937, -0.004037084301382362454, -0.2362204724409449064 ) ) ;
#11085=CARTESIAN_POINT ( 'NONE',  ( -0.7246715730664488042, 0.2211122077665220453, 0.05732876522465197439 ) ) ;
#11087=ORIENTED_EDGE ( 'NONE', *, *, #26541, .T. ) ;
#11114=CARTESIAN_POINT ( 'NONE',  ( 0.3334645669291338987, -0.8041772776331653771, -0.9118913923173522784 ) ) ;
#11127=CARTESIAN_POINT ( 'NONE',  ( 0.7640955261426980449, 0.5878663239606607416, 0.09435744292894028551 ) ) ;
#11150=CARTESIAN_POINT ( 'NONE',  ( -0.4169216294785028087, -0.5582982840830001958, -0.4568332836680285003 ) ) ;
#11184=ADVANCED_FACE ( 'NONE', ( #10772 ), #23512, .T. ) ;
#11213=CARTESIAN_POINT ( 'NONE',  ( -0.7246715730664488042, 0.1595564285404119931, -0.2516711161248811335 ) ) ;
#11276=CARTESIAN_POINT ( 'NONE',  ( -0.3614376061968875287, -1.111631388898730588, -0.4004058270235824613 ) ) ;
#11280=FACE_OUTER_BOUND ( 'NONE', #27389, .T. ) ;
#11306=FACE_OUTER_BOUND ( 'NONE', #1631, .T. ) ;
#11326=CARTESIAN_POINT ( 'NONE',  ( 0.7874015748031325534, 0.2476103627152109743, -0.2796030453571548002 ) ) ;
#11346=LINE ( 'NONE', #20382, #6561 ) ;
#11356=CARTESIAN_POINT ( 'NONE',  ( -0.6562077975700097987, -7.454212598425196280E-14, -0.07874015748031495954 ) ) ;
#11362=DIRECTION ( 'NONE',  ( 1.000000000000000000, 0.000000000000000000, 0.000000000000000000 ) ) ;
#11398=CARTESIAN_POINT ( 'NONE',  ( 0.6933858814654041414, 0.7755322313789173583, -0.02322279011146228048 ) ) ;
#11458=CIRCLE ( 'NONE', #8748, 1.288838582677165112 ) ;
#11482=CARTESIAN_POINT ( 'NONE',  ( -0.6562077975700453258, 1.655117322834645733E-14, -0.2362204724409449064 ) ) ;
#11491=CARTESIAN_POINT ( 'NONE',  ( -0.7874015748031496509, 0.3648237195092146057, -0.1496552535541220419 ) ) ;
#11520=CARTESIAN_POINT ( 'NONE',  ( -0.7874015748031496509, 0.3648237195092146057, -0.1496552535541220419 ) ) ;
#11533=CARTESIAN_POINT ( 'NONE',  ( 0.2083728861314909642, 0.5965552328248759917, 0.1367407604580403446 ) ) ;
#11551=ORIENTED_EDGE ( 'NONE', *, *, #9655, .F. ) ;
#11560=ORIENTED_EDGE ( 'NONE', *, *, #20508, .T. ) ;
#11564=DIRECTION ( 'NONE',  ( 1.000000000000000000, 0.000000000000000000, 0.000000000000000000 ) ) ;
#11573=FACE_OUTER_BOUND ( 'NONE', #18417, .T. ) ;
#11584=DIRECTION ( 'NONE',  ( -1.000000000000000000, 0.000000000000000000, 0.000000000000000000 ) ) ;
#11588=AXIS2_PLACEMENT_3D ( 'NONE', #5229, #3665, #7923 ) ;
#11592=EDGE_LOOP ( 'NONE', ( #7743, #801, #27491, #1286 ) ) ;
#11598=CARTESIAN_POINT ( 'NONE',  ( 0.6175000359513720394, 0.7947887377729331293, -0.2396602654345149352 ) ) ;
#11648=CARTESIAN_POINT ( 'NONE',  ( -0.7432982829791772161, 0.2032415433700952845, -0.2614846436432287091 ) ) ;
#11652=CARTESIAN_POINT ( 'NONE',  ( -0.3681444341728476455, -1.081405805935157449, -0.3462526684107952724 ) ) ;
#11664=CARTESIAN_POINT ( 'NONE',  ( -0.3609634007533684685, -0.7054839598378710441, -0.6417682067245982225 ) ) ;
#11671=CARTESIAN_POINT ( 'NONE',  ( -0.1786951194748074845, 1.156667798187631879, -0.4648257047102559159 ) ) ;
#11675=CARTESIAN_POINT ( 'NONE',  ( 0.5620070256527415209, 0.9643919186718870051, -0.1975661767702522054 ) ) ;
#11698=ORIENTED_EDGE ( 'NONE', *, *, #1223, .F. ) ;
#11706=LINE ( 'NONE', #5402, #2001 ) ;
#11734=DIRECTION ( 'NONE',  ( -1.000000000000000000, 0.000000000000000000, 0.000000000000000000 ) ) ;
#11741=CARTESIAN_POINT ( 'NONE',  ( 0.7873253891977465280, 0.2508138056050463471, -0.2773433314823283702 ) ) ;
#11802=ADVANCED_FACE ( 'NONE', ( #24797 ), #20145, .T. ) ;
#11833=AXIS2_PLACEMENT_3D ( 'NONE', #20720, #5761, #20859 ) ;
#11881=CARTESIAN_POINT ( 'NONE',  ( 0.5309636003393858328, 0.7559193067387677267, -0.4362061884873984496 ) ) ;
#11905=CARTESIAN_POINT ( 'NONE',  ( 0.1819818857492424280, 0.6289820519968024604, 0.07987519446618293606 ) ) ;
#11919=CARTESIAN_POINT ( 'NONE',  ( 0.3334645669291338987, 0.000000000000000000, -1.052618110236220428 ) ) ;
#11935=EDGE_CURVE ( 'NONE', #3730, #15240, #14662, .T. ) ;
#11950=CARTESIAN_POINT ( 'NONE',  ( 0.04115487667019134682, -0.6180305271469684891, 0.08832868324785138336 ) ) ;
#11953=CARTESIAN_POINT ( 'NONE',  ( -0.4307861782378184512, -0.5235511812839959145, -0.4261998249987570264 ) ) ;
#11956=ORIENTED_EDGE ( 'NONE', *, *, #7820, .T. ) ;
#11957=EDGE_LOOP ( 'NONE', ( #10463, #5502, #21452, #18584 ) ) ;
#11964=CARTESIAN_POINT ( 'NONE',  ( 0.5530354143091553709, 0.9746577485994293299, -0.2092867075132898436 ) ) ;
#11965=CARTESIAN_POINT ( 'NONE',  ( 0.7874015748031496509, 3.035194737559055338E-06, -1.475314960619023674 ) ) ;
#11972=CARTESIAN_POINT ( 'NONE',  ( 0.5890517850735842442, -0.1332273157280143838, -0.2362204724409449064 ) ) ;
#11987=CARTESIAN_POINT ( 'NONE',  ( 0.3339160553493882300, 0.7867001919223544082, -0.8344257386302499357 ) ) ;
#12028=LINE ( 'NONE', #1296, #17049 ) ;
#12040=B_SPLINE_SURFACE_WITH_KNOTS ( 'NONE', 3, 3, ( 
 ( #24047, #5242, #22199, #1018, #13861, #7096, #11326 ),
 ( #19945, #22062, #7365, #15713, #11741, #26854, #15986 ),
 ( #22340, #17934, #20081, #24315, #599, #22484, #20222 ),
 ( #5393, #14013, #26297, #7221, #9192, #2824, #4963 ),
 ( #15840, #736, #26430, #9610, #13577, #9325, #22623 ),
 ( #13436, #2965, #17811, #24444, #24590, #2692, #3112 ),
 ( #18217, #11598, #7507, #26565, #5094, #20503, #9467 ),
 ( #13717, #4820, #11881, #18064, #16133, #26706, #24732 ),
 ( #3243, #9063, #17677, #6963, #15585, #24189, #8081 ) ),
 .UNSPECIFIED., .F., .F., .F.,
 ( 4, 3, 1, 1, 4 ),
 ( 4, 3, 4 ),
 ( -0.9890658252508724990, -0.9807067265327750194, -0.6976453139676740411, -0.5089377055909399816, -0.3202300972142069768 ),
 ( 0.000000000000000000, 1.199999999999999956, 1.211999999999999966 ),
 .UNSPECIFIED. ) ;
#12044=CARTESIAN_POINT ( 'NONE',  ( 0.4563908000638740581, 0.6818102780177048849, -0.6021022548816948872 ) ) ;
#12075=CARTESIAN_POINT ( 'NONE',  ( -0.4101012214746874163, -0.5753751194595236873, -0.4717551279267843123 ) ) ;
#12100=CARTESIAN_POINT ( 'NONE',  ( -0.2490711204941342405, 0.9131938423895413770, -0.7142170566240019225 ) ) ;
#12109=CARTESIAN_POINT ( 'NONE',  ( 0.5890517850735833560, -0.2103183229436192403, 0.2232855712133572090 ) ) ;
#12117=CARTESIAN_POINT ( 'NONE',  ( -0.3334645669291338987, 0.8103892183150610551, -0.9220603341868013336 ) ) ;
#12139=CARTESIAN_POINT ( 'NONE',  ( -0.6042317347120136350, -0.1855048251218045230, 0.2228014207307441874 ) ) ;
#12145=ORIENTED_EDGE ( 'NONE', *, *, #24591, .T. ) ;
#12227=CARTESIAN_POINT ( 'NONE',  ( -0.6065227633320124934, -0.1124154687194963698, -0.2439881145186360845 ) ) ;
#12243=FACE_OUTER_BOUND ( 'NONE', #23904, .T. ) ;
#12259=CARTESIAN_POINT ( 'NONE',  ( 0.3611077606078542668, 0.7441461625961331983, -0.7153708716273008417 ) ) ;
#12283=CARTESIAN_POINT ( 'NONE',  ( -0.4326303163632846394, -0.8192757351588600967, -0.05768471019755529866 ) ) ;
#12318=EDGE_LOOP ( 'NONE', ( #17872, #13213, #10063, #27416 ) ) ;
#12339=CARTESIAN_POINT ( 'NONE',  ( 0.7874015748031496509, -0.4579607000970866149, -0.1931355542581366103 ) ) ;
#12356=CARTESIAN_POINT ( 'NONE',  ( -0.5935113537020059171, -0.1684283806775520032, -0.09332418187737165360 ) ) ;
#12367=CARTESIAN_POINT ( 'NONE',  ( -0.4612762626262458809, -0.4482319504133971400, -0.3686284328691009637 ) ) ;
#12406=CARTESIAN_POINT ( 'NONE',  ( 0.3393484408203505942, 0.7678314947796125445, -0.7734693920224366970 ) ) ;
#12430=CARTESIAN_POINT ( 'NONE',  ( -0.4386012532733669644, -0.7958710277660615562, -0.03879670081233077550 ) ) ;
#12439=SHAPE_REPRESENTATION_RELATIONSHIP ( 'NONE' , 'NONE' ,  #19852, #24825 ) ;
#12457=CARTESIAN_POINT ( 'NONE',  ( 0.7874015748031151229, 0.2490421840548274757, -0.2751330019808225780 ) ) ;
#12500=CARTESIAN_POINT ( 'NONE',  ( -0.6002615430280354714, -0.1993712550749956736, 0.2207846809961432899 ) ) ;
#12508=B_SPLINE_SURFACE_WITH_KNOTS ( 'NONE', 3, 3, ( 
 ( #2100, #15395, #27819, #23986 ),
 ( #8456, #17079, #6625, #25695 ),
 ( #10996, #4621, #19619, #15249 ),
 ( #8865, #2506, #12832, #34 ) ),
 .UNSPECIFIED., .F., .F., .F.,
 ( 4, 4 ),
 ( 4, 4 ),
 ( -0.3202300972144559998, -0.1691655120378159904 ),
 ( -4.440891999999999804E-16, 1.199999999999999956 ),
 .UNSPECIFIED. ) ;
#12541=EDGE_LOOP ( 'NONE', ( #18549, #26598, #10131, #2098, #4414 ) ) ;
#12588=LINE ( 'NONE', #10039, #20825 ) ;
#12620=VERTEX_POINT ( 'NONE', #23670 ) ;
#12623=CARTESIAN_POINT ( 'NONE',  ( -0.7874015748031496509, 0.4828108945773819105, 0.1423708153504031348 ) ) ;
#12636=CARTESIAN_POINT ( 'NONE',  ( -0.5355664161054535244, -0.3771716564148893669, 0.01418171057387437005 ) ) ;
#12639=AXIS2_PLACEMENT_3D ( 'NONE', #6825, #21939, #13311 ) ;
#12645=CARTESIAN_POINT ( 'NONE',  ( 0.1120675189988346587, -0.7410715175625038897, 0.001857066358701141805 ) ) ;
#12649=CARTESIAN_POINT ( 'NONE',  ( -0.6104814441609700548, -0.1036450511418069570, -0.2428261403048069811 ) ) ;
#12668=CARTESIAN_POINT ( 'NONE',  ( -0.4359497604187455577, 0.2332958656722624868, -0.2680411597722005546 ) ) ;
#12687=CARTESIAN_POINT ( 'NONE',  ( -0.2490711204941346568, 0.7655264129003995777, -0.7689379837741201484 ) ) ;
#12700=CARTESIAN_POINT ( 'NONE',  ( -0.5942349471504173586, -0.2203927747844337814, 0.2172369878168960988 ) ) ;
#12763=DIRECTION ( 'NONE',  ( 1.000000000000000000, 0.000000000000000000, 0.000000000000000000 ) ) ;
#12772=CARTESIAN_POINT ( 'NONE',  ( -0.4995226175161708859, -0.4253379528844141721, -0.1763862759506159561 ) ) ;
#12802=CARTESIAN_POINT ( 'NONE',  ( -0.3334645669291338987, 9.254566434606299706E-06, -2.341456692880161228 ) ) ;
#12806=CIRCLE ( 'NONE', #7838, 1.288838582677165556 ) ;
#12807=CARTESIAN_POINT ( 'NONE',  ( -0.2602238532265429005, 0.000000000000000000, -0.2362204724409449064 ) ) ;
#12817=CARTESIAN_POINT ( 'NONE',  ( 0.3561571326799479742, 1.175382753584212514, -0.5166459152402519406 ) ) ;
#12821=ORIENTED_EDGE ( 'NONE', *, *, #14034, .T. ) ;
#12828=CARTESIAN_POINT ( 'NONE',  ( -0.1786951194748074845, 0.7326758143707651216, -0.6802888381025230524 ) ) ;
#12832=CARTESIAN_POINT ( 'NONE',  ( 0.3976891862754212137, 0.8566358266442657410, -0.5893543329197449276 ) ) ;
#12856=CARTESIAN_POINT ( 'NONE',  ( -0.6562077975700374433, -2.731848031496062854E-17, 0.1574803149606299191 ) ) ;
#12873=CARTESIAN_POINT ( 'NONE',  ( 0.3334645669291338987, -0.7876517371453680694, -0.8174568431611989316 ) ) ;
#12909=AXIS2_PLACEMENT_3D ( 'NONE', #27597, #6404, #21785 ) ;
#12910=CARTESIAN_POINT ( 'NONE',  ( -0.5252801253069795395, -0.2960335176359168985, -0.2916644167427649981 ) ) ;
#12915=ADVANCED_FACE ( 'NONE', ( #11573 ), #27223, .T. ) ;
#12918=CARTESIAN_POINT ( 'NONE',  ( -0.7432982829791772161, 0.2424461424275303201, -0.1088776918758622148 ) ) ;
#12951=ADVANCED_FACE ( 'NONE', ( #12243 ), #22174, .F. ) ;
#12975=CARTESIAN_POINT ( 'NONE',  ( -0.3613813581019308385, -1.111881281712430614, -0.4008318706050917335 ) ) ;
#12979=CYLINDRICAL_SURFACE ( 'NONE', #23228, 0.8163976377952756325 ) ;
#12983=PRODUCT_DEFINITION_FORMATION_WITH_SPECIFIED_SOURCE ( 'ANY', '', #23113, .NOT_KNOWN. ) ;
#12985=( LENGTH_UNIT ( ) NAMED_UNIT ( * ) SI_UNIT ( $, .METRE. ) ) ;
#13001=DIRECTION ( 'NONE',  ( 0.000000000000000000, 0.000000000000000000, 1.000000000000000000 ) ) ;
#13015=CYLINDRICAL_SURFACE ( 'NONE', #23667, 1.288838582677165556 ) ;
#13017=LINE ( 'NONE', #23636, #6966 ) ;
#13104=ORIENTED_EDGE ( 'NONE', *, *, #19932, .T. ) ;
#13145=ORIENTED_EDGE ( 'NONE', *, *, #10157, .T. ) ;
#13152=EDGE_CURVE ( 'NONE', #13674, #24360, #10962, .T. ) ;
#13164=CARTESIAN_POINT ( 'NONE',  ( 0.3102399269716953345, -1.154980647406259830, -0.4411320940076480235 ) ) ;
#13200=CARTESIAN_POINT ( 'NONE',  ( -0.2602238532265429005, 0.000000000000000000, -0.07874015748031495954 ) ) ;
#13213=ORIENTED_EDGE ( 'NONE', *, *, #22280, .F. ) ;
#13247=CARTESIAN_POINT ( 'NONE',  ( 0.7864367829959311162, 0.4380964431885162602, 0.1600151387865518249 ) ) ;
#13256=CARTESIAN_POINT ( 'NONE',  ( -0.8725268807032540153, 0.000000000000000000, -1.052618110236220428 ) ) ;
#13261=CARTESIAN_POINT ( 'NONE',  ( -0.8725268807032540153, 0.000000000000000000, -1.052618110236220428 ) ) ;
#13311=DIRECTION ( 'NONE',  ( 0.000000000000000000, -7.180547322999999937E-06, -0.9999999999742198442 ) ) ;
#13328=CARTESIAN_POINT ( 'NONE',  ( -0.6505662911506299162, -0.01296944263642094489, -0.2362868447687200835 ) ) ;
#13338=ORIENTED_EDGE ( 'NONE', *, *, #6493, .T. ) ;
#13365=CARTESIAN_POINT ( 'NONE',  ( 0.1532705055535415473, -0.5147072688414000563, -0.4165008336377047371 ) ) ;
#13381=CARTESIAN_POINT ( 'NONE',  ( 0.7529539909399990405, 0.6316670891464889470, 0.07132544462029670462 ) ) ;
#13387=CARTESIAN_POINT ( 'NONE',  ( -0.3666422121843372350, -1.088756306996242484, -0.3628375440173792765 ) ) ;
#13436=CARTESIAN_POINT ( 'NONE',  ( 0.7430739993161732393, 0.7025059129074271436, 0.04061420537818291598 ) ) ;
#13456=CARTESIAN_POINT ( 'NONE',  ( -0.6208708315385689236, -0.09594997026702008214, -0.08344808172604054053 ) ) ;
#13465=CARTESIAN_POINT ( 'NONE',  ( -0.6587140840999922142, 0.005767656754036574844, -0.2362204724409449064 ) ) ;
#13468=LINE ( 'NONE', #10812, #17446 ) ;
#13499=EDGE_LOOP ( 'NONE', ( #686, #16710, #19083, #26892 ) ) ;
#13563=ORIENTED_EDGE ( 'NONE', *, *, #13942, .F. ) ;
#13577=CARTESIAN_POINT ( 'NONE',  ( 0.7845931698711713365, 0.3312401467028460722, -0.3038783524521976309 ) ) ;
#13595=CARTESIAN_POINT ( 'NONE',  ( -0.6165893942483189338, -0.09003804048641948776, -0.2411755456731409508 ) ) ;
#13610=EDGE_LOOP ( 'NONE', ( #557, #26232, #25961, #13338 ) ) ;
#13626=CARTESIAN_POINT ( 'NONE',  ( -0.6996199877990079141, 0.1008405537593297374, -0.2423665665178251771 ) ) ;
#13674=VERTEX_POINT ( 'NONE', #8771 ) ;
#13700=DIRECTION ( 'NONE',  ( 0.000000000000000000, 0.9636237974020582797, 0.2672623749809110993 ) ) ;
#13717=CARTESIAN_POINT ( 'NONE',  ( 0.5309636003393858328, 1.000390209383793305, -0.2368508997780850722 ) ) ;
#13723=ORIENTED_EDGE ( 'NONE', *, *, #14242, .T. ) ;
#13745=CARTESIAN_POINT ( 'NONE',  ( 0.3976891862754212137, 0.9951575781684135480, -0.5144425584461574941 ) ) ;
#13750=DIRECTION ( 'NONE',  ( 1.000000000000000000, 0.000000000000000000, 0.000000000000000000 ) ) ;
#13760=CARTESIAN_POINT ( 'NONE',  ( 0.1120675189988346587, -0.4694218845611126678, -0.3846748511993476338 ) ) ;
#13782=CARTESIAN_POINT ( 'NONE',  ( 0.7874015748031496509, 0.3810512208497282005, 0.1369858506767638040 ) ) ;
#13792=ORIENTED_EDGE ( 'NONE', *, *, #15166, .F. ) ;
#13793=EDGE_LOOP ( 'NONE', ( #16504, #37, #6988, #24058 ) ) ;
#13823=ORIENTED_EDGE ( 'NONE', *, *, #14612, .T. ) ;
#13835=DIRECTION ( 'NONE',  ( -1.000000000000000000, 0.000000000000000000, 0.000000000000000000 ) ) ;
#13854=ORIENTED_EDGE ( 'NONE', *, *, #23037, .T. ) ;
#13861=CARTESIAN_POINT ( 'NONE',  ( 0.7874015748031325534, 0.2485711856858030810, -0.2766034250564945451 ) ) ;
#13891=VERTEX_POINT ( 'NONE', #8336 ) ;
#13915=VECTOR ( 'NONE', #2706, 39.37007874015748143 ) ;
#13918=CARTESIAN_POINT ( 'NONE',  ( -0.6562077975700374433, -1.365924015748031427E-17, -0.2362204724409449064 ) ) ;
#13920=CARTESIAN_POINT ( 'NONE',  ( -0.3681444341728476455, -0.8171366637306790581, -0.5188711171093385310 ) ) ;
#13925=CARTESIAN_POINT ( 'NONE',  ( 0.7874015748031497619, 0.3689420268555997362, 0.09918206336684766422 ) ) ;
#13930=CARTESIAN_POINT ( 'NONE',  ( -0.3430084144618599784, -0.7594774848350865915, -0.7521500857743448343 ) ) ;
#13933=DIRECTION ( 'NONE',  ( 0.000000000000000000, 0.000000000000000000, 1.000000000000000000 ) ) ;
#13940=B_SPLINE_CURVE_WITH_KNOTS ( 'NONE', 3,
 ( #1233, #20149, #9831, #16203, #16339, #26783, #7431, #805, #5463, #18000, #16060, #26639, #7295 ),
 .UNSPECIFIED., .F., .F.,
 ( 4, 1, 1, 1, 1, 1, 1, 1, 1, 1, 4 ),
 ( -0.4911627496483090272, -0.4713348141022760118, -0.4508419969318550047, -0.4405955883466449730, -0.4252259754688289539, -0.4201027711762239658, -0.4098563625910129904, -0.4047331582984080023, -0.3944867497131970269, -0.3893635454205919832, -0.3833360769390280476 ),
 .UNSPECIFIED. ) ;
#13942=EDGE_CURVE ( 'NONE', #527, #6591, #12806, .T. ) ;
#13960=VECTOR ( 'NONE', #7742, 39.37007874015748143 ) ;
#13961=CARTESIAN_POINT ( 'NONE',  ( 0.4898768902087983768, 0.000000000000000000, 0.2362204724409449064 ) ) ;
#13963=EDGE_LOOP ( 'NONE', ( #10961, #23980, #6951, #945, #2451 ) ) ;
#13986=CARTESIAN_POINT ( 'NONE',  ( -0.8725268807032540153, 0.000000000000000000, 0.2362204724409449619 ) ) ;
#14013=CARTESIAN_POINT ( 'NONE',  ( 0.7871730179869745880, 0.3544754436444846335, 0.02177413181674842796 ) ) ;
#14029=DIRECTION ( 'NONE',  ( 0.000000000000000000, -0.8089354696471389161, -0.5878974450929028706 ) ) ;
#14034=EDGE_CURVE ( 'NONE', #13674, #3730, #6486, .T. ) ;
#14049=ORIENTED_EDGE ( 'NONE', *, *, #8536, .F. ) ;
#14058=CARTESIAN_POINT ( 'NONE',  ( -0.7874015748031496509, 0.3058301319751310920, -0.2956682880063846164 ) ) ;
#14074=CARTESIAN_POINT ( 'NONE',  ( -0.4134148064934505262, -0.5671632014791846421, -0.4652690387879091505 ) ) ;
#14128=EDGE_CURVE ( 'NONE', #16084, #6657, #19628, .T. ) ;
#14134=CARTESIAN_POINT ( 'NONE',  ( -0.6098077518716100709, -0.1659937022319242506, 0.2254863467269558330 ) ) ;
#14161=CARTESIAN_POINT ( 'NONE',  ( 0.7873254110087903879, 0.2512946835069670426, -0.2758545172576901128 ) ) ;
#14213=CARTESIAN_POINT ( 'NONE',  ( -0.3338887748335570560, -1.114136943608293295, -0.8559701994470926278 ) ) ;
#14225=B_SPLINE_CURVE_WITH_KNOTS ( 'NONE', 3,
 ( #469, #351, #17005, #13164, #2164, #8930 ),
 .UNSPECIFIED., .F., .F.,
 ( 4, 1, 1, 4 ),
 ( 0.000000000000000000, 0.2857142857142859760, 0.5714285714285719520, 1.000000000000000000 ),
 .UNSPECIFIED. ) ;
#14242=EDGE_CURVE ( 'NONE', #550, #15744, #5564, .T. ) ;
#14245=ADVANCED_FACE ( 'NONE', ( #9407 ), #18011, .T. ) ;
#14282=CARTESIAN_POINT ( 'NONE',  ( -0.5656894121276926368, -0.3210335855601377797, 0.1956008235395614858 ) ) ;
#14298=CARTESIAN_POINT ( 'NONE',  ( -0.8725268807032540153, 0.000000000000000000, -1.052618110236220428 ) ) ;
#14306=VECTOR ( 'NONE', #26841, 39.37007874015748143 ) ;
#14313=CARTESIAN_POINT ( 'NONE',  ( 0.3976891862754212137, 0.7181140751201200434, -0.6642661073933326943 ) ) ;
#14333=EDGE_LOOP ( 'NONE', ( #27526, #24628, #22831 ) ) ;
#14338=CARTESIAN_POINT ( 'NONE',  ( 0.7874015748031496509, -0.6060691875862775913, 0.08482860590295551728 ) ) ;
#14354=ORIENTED_EDGE ( 'NONE', *, *, #17265, .F. ) ;
#14359=LINE ( 'NONE', #7718, #7305 ) ;
#14364=CARTESIAN_POINT ( 'NONE',  ( -0.3602580257949353215, -0.7074757604431674007, -0.6452024007641304904 ) ) ;
#14379=CARTESIAN_POINT ( 'NONE',  ( -0.7874015748031496509, -5.862181872598426086E-06, -1.869015748010449007 ) ) ;
#14405=CARTESIAN_POINT ( 'NONE',  ( 0.3976891862754212137, 0.7181140751201200434, -0.6642661073933326943 ) ) ;
#14426=CARTESIAN_POINT ( 'NONE',  ( -0.5365253175192220558, -0.4262145198643368937, 0.1637104082999795707 ) ) ;
#14501=CARTESIAN_POINT ( 'NONE',  ( -0.5833277509429386498, -0.1953566107329901547, -0.09839827897590196215 ) ) ;
#14512=CARTESIAN_POINT ( 'NONE',  ( 0.04115487667019134682, -0.5425147539706086652, -0.05108106348549787401 ) ) ;
#14515=CARTESIAN_POINT ( 'NONE',  ( -0.6187410091539320423, -0.08521673449347196005, -0.2406752346771077189 ) ) ;
#14540=CARTESIAN_POINT ( 'NONE',  ( 0.6882266799383695011, -0.4143730867902977177, 0.1723141108463512317 ) ) ;
#14577=CARTESIAN_POINT ( 'NONE',  ( -0.5885963067485330269, -0.2400798436957021775, 0.2138130534390355331 ) ) ;
#14612=EDGE_CURVE ( 'NONE', #607, #22369, #7853, .T. ) ;
#14638=CARTESIAN_POINT ( 'NONE',  ( 0.7874015748031496509, 0.000000000000000000, -1.052618110236220428 ) ) ;
#14647=CARTESIAN_POINT ( 'NONE',  ( -0.4881018399981850719, -0.3837266214674216469, -0.3317898348603995351 ) ) ;
#14662=LINE ( 'NONE', #5891, #8599 ) ;
#14693=ORIENTED_EDGE ( 'NONE', *, *, #2713, .T. ) ;
#14725=CARTESIAN_POINT ( 'NONE',  ( -0.5943649339014159816, -0.2199389736434831377, 0.2173156648486553322 ) ) ;
#14791=CARTESIAN_POINT ( 'NONE',  ( -0.6068752646683485130, -0.1331980723927974342, -0.08786100608780256227 ) ) ;
#14794=ORIENTED_EDGE ( 'NONE', *, *, #4995, .F. ) ;
#14803=CARTESIAN_POINT ( 'NONE',  ( -0.5551587109978235457, -0.2272353400451556926, -0.2684417395417463270 ) ) ;
#14807=CARTESIAN_POINT ( 'NONE',  ( -0.3355349563089153886, 0.1206850104808647739, -0.07874015748031495954 ) ) ;
#14827=EDGE_CURVE ( 'NONE', #18714, #6657, #13017, .T. ) ;
#14832=CARTESIAN_POINT ( 'NONE',  ( 0.3976891862754212137, 0.7181140751201181560, -0.6642661073933326943 ) ) ;
#14851=CARTESIAN_POINT ( 'NONE',  ( -0.5427308778234085640, -0.4036295907641927472, 0.1714462237544466250 ) ) ;
#14852=CARTESIAN_POINT ( 'NONE',  ( 0.3334645669291338987, -5.862181872992126152E-06, -1.869015748010449007 ) ) ;
#14912=VECTOR ( 'NONE', #15490, 39.37007874015748143 ) ;
#14922=CARTESIAN_POINT ( 'NONE',  ( -0.5355664161054535244, -0.2721702372959802774, -0.2828063903444661409 ) ) ;
#14937=CARTESIAN_POINT ( 'NONE',  ( -0.5298607097989774806, -0.2854075319011052381, -0.2877231093509545201 ) ) ;
#14964=CARTESIAN_POINT ( 'NONE',  ( 0.3976891862754212137, 0.8566358266442657410, -0.5893543329197449276 ) ) ;
#14998=FACE_OUTER_BOUND ( 'NONE', #26073, .T. ) ;
#15007=CARTESIAN_POINT ( 'NONE',  ( -0.8725268807032540153, 0.000000000000000000, -1.052618110236220428 ) ) ;
#15036=CARTESIAN_POINT ( 'NONE',  ( -0.1361267291514174083, -0.1666946003182495917, -0.2490847877778887554 ) ) ;
#15041=DIRECTION ( 'NONE',  ( 0.000000000000000000, 7.180547322999998243E-06, -0.9999999999742198442 ) ) ;
#15057=CARTESIAN_POINT ( 'NONE',  ( -0.5632721120450597807, -0.2087920062485354444, -0.2632549038600744407 ) ) ;
#15068=CARTESIAN_POINT ( 'NONE',  ( -0.7121770198535963825, 0.2056174084053519757, 0.2200249214779901596 ) ) ;
#15071=CARTESIAN_POINT ( 'NONE',  ( -0.5317387256069298074, -0.2810540235075434379, -0.2861221005886522284 ) ) ;
#15074=CARTESIAN_POINT ( 'NONE',  ( -0.3355349563089153886, 0.1011697176171429124, -0.2362204724409449064 ) ) ;
#15101=CARTESIAN_POINT ( 'NONE',  ( 0.3102399269716953345, -0.7316071111737637578, -0.6652804359117283628 ) ) ;
#15142=ORIENTED_EDGE ( 'NONE', *, *, #7364, .F. ) ;
#15166=EDGE_CURVE ( 'NONE', #25001, #18714, #21043, .T. ) ;
#15179=CARTESIAN_POINT ( 'NONE',  ( 0.4895462770359960136, 1.042587244177305195, -0.2949132003431571003 ) ) ;
#15187=CARTESIAN_POINT ( 'NONE',  ( -0.6562077975700453258, 1.974383858267716320E-14, -0.07874015748031495954 ) ) ;
#15199=CARTESIAN_POINT ( 'NONE',  ( -0.6722178168900768691, 0.05837462721528850068, 0.2350617247236460594 ) ) ;
#15214=CARTESIAN_POINT ( 'NONE',  ( -0.2490711204941346568, 0.7655264129003995777, -0.7689379837741201484 ) ) ;
#15215=ORIENTED_EDGE ( 'NONE', *, *, #10157, .F. ) ;
#15240=VERTEX_POINT ( 'NONE', #21473 ) ;
#15249=CARTESIAN_POINT ( 'NONE',  ( 0.4245040230929275626, 0.7010584879323878971, -0.6327280771288050776 ) ) ;
#15318=CARTESIAN_POINT ( 'NONE',  ( 0.7874015748031496509, 3.035194737716535704E-06, -1.475314960619023674 ) ) ;
#15358=CARTESIAN_POINT ( 'NONE',  ( 0.3102399269716953345, -1.154980647406259830, -0.4411320940076480235 ) ) ;
#15362=CARTESIAN_POINT ( 'NONE',  ( 0.7874015748031496509, 0.000000000000000000, -1.052618110236220428 ) ) ;
#15367=ADVANCED_FACE ( 'NONE', ( #4511 ), #12979, .T. ) ;
#15395=CARTESIAN_POINT ( 'NONE',  ( 0.4895462770359960136, 0.9151958316344488420, -0.3874954751609366310 ) ) ;
#15397=CARTESIAN_POINT ( 'NONE',  ( 0.6141002140709024282, 0.8998311997009023067, -0.1298280283246295574 ) ) ;
#15439=CARTESIAN_POINT ( 'NONE',  ( 0.4898768902087983768, 0.000000000000000000, -0.2362204724409449064 ) ) ;
#15445=CARTESIAN_POINT ( 'NONE',  ( -0.3338887748335570560, -1.036595354089161480, -0.8696564807123209340 ) ) ;
#15456=VERTEX_POINT ( 'NONE', #23335 ) ;
#15466=ORIENTED_EDGE ( 'NONE', *, *, #19409, .T. ) ;
#15467=CARTESIAN_POINT ( 'NONE',  ( -0.6208708315385689236, -0.1114655006168945028, 0.07327095640358681494 ) ) ;
#15479=CARTESIAN_POINT ( 'NONE',  ( -0.6806799598997224088, 0.05663649493104071925, -0.2380830294301988226 ) ) ;
#15483=DIRECTION ( 'NONE',  ( 1.000000000000000000, 0.000000000000000000, 0.000000000000000000 ) ) ;
#15490=DIRECTION ( 'NONE',  ( 0.000000000000000000, 0.000000000000000000, -1.000000000000000000 ) ) ;
#15509=ORIENTED_EDGE ( 'NONE', *, *, #14128, .F. ) ;
#15514=ORIENTED_EDGE ( 'NONE', *, *, #1754, .F. ) ;
#15536=CIRCLE ( 'NONE', #1990, 1.288838582677165778 ) ;
#15585=CARTESIAN_POINT ( 'NONE',  ( 0.4895462770358314786, 0.6591390924234138415, -0.5735858475448201155 ) ) ;
#15614=CARTESIAN_POINT ( 'NONE',  ( -0.6587140840999922142, 0.009105340598872481081, 0.2362204724409449064 ) ) ;
#15625=DIRECTION ( 'NONE',  ( 0.000000000000000000, 0.9376881772560526906, 0.3474778874032439235 ) ) ;
#15655=CARTESIAN_POINT ( 'NONE',  ( 0.6995334740348704283, 0.7637040338457791178, -0.01440115984997634123 ) ) ;
#15659=CARTESIAN_POINT ( 'NONE',  ( 0.7874015748031496509, -5.862181872755905604E-06, -1.869015748010449007 ) ) ;
#15704=FACE_OUTER_BOUND ( 'NONE', #13963, .T. ) ;
#15713=CARTESIAN_POINT ( 'NONE',  ( 0.7873253891977465280, 0.2512985515673845649, -0.2758449551032512992 ) ) ;
#15732=CARTESIAN_POINT ( 'NONE',  ( -0.6165893942483189338, -0.1247741027201273722, 0.07187346404476555040 ) ) ;
#15744=VERTEX_POINT ( 'NONE', #8574 ) ;
#15748=CARTESIAN_POINT ( 'NONE',  ( -0.5112608635011182123, 0.5325127325997165428, 0.1663800295771515891 ) ) ;
#15783=CARTESIAN_POINT ( 'NONE',  ( -0.2490711204941342405, 0.9131938423895413770, -0.7142170566240019225 ) ) ;
#15789=DIRECTION ( 'NONE',  ( 1.000000000000000000, 0.000000000000000000, 0.000000000000000000 ) ) ;
#15825=CARTESIAN_POINT ( 'NONE',  ( -0.6266852695743893031, -0.1062821802600274479, 0.2318330448317133807 ) ) ;
#15840=CARTESIAN_POINT ( 'NONE',  ( 0.7845931698711713365, 0.5239360887457676919, 0.1316939677558954802 ) ) ;
#15874=EDGE_CURVE ( 'NONE', #12620, #10641, #11346, .T. ) ;
#15893=CARTESIAN_POINT ( 'NONE',  ( -0.3338887748335567229, -1.104088614729972440, -0.7990416445823268488 ) ) ;
#15915=CARTESIAN_POINT ( 'NONE',  ( 0.2083728861314909642, 0.3778799683983641300, -0.2992345713071495883 ) ) ;
#15917=CARTESIAN_POINT ( 'NONE',  ( 0.4895462770359960136, 1.042587244177305195, -0.2949132003431571003 ) ) ;
#15984=ORIENTED_EDGE ( 'NONE', *, *, #1223, .T. ) ;
#15986=CARTESIAN_POINT ( 'NONE',  ( 0.7873253891977465280, 0.2498443136803698561, -0.2803400842404824567 ) ) ;
#16031=ORIENTED_EDGE ( 'NONE', *, *, #24591, .F. ) ;
#16040=CARTESIAN_POINT ( 'NONE',  ( -0.3861436020174326966, -1.005626036844328830, -0.2420500664475239982 ) ) ;
#16049=CARTESIAN_POINT ( 'NONE',  ( 0.7874015748031496509, 0.2607538277840750762, -0.2385700914728043909 ) ) ;
#16050=CARTESIAN_POINT ( 'NONE',  ( -0.2602238532265429005, 0.000000000000000000, 0.2362204724409449064 ) ) ;
#16053=CARTESIAN_POINT ( 'NONE',  ( -0.3611053385039311725, -0.7050837974523566087, -0.6410818428499839294 ) ) ;
#16060=CARTESIAN_POINT ( 'NONE',  ( -0.6633461167951516524, 0.02596910924942653909, 0.2360419752028775631 ) ) ;
#16061=LINE ( 'NONE', #24655, #25286 ) ;
#16063=CARTESIAN_POINT ( 'NONE',  ( 0.2083728861314909642, 0.4507717232072007696, -0.1539094607187527497 ) ) ;
#16065=DIRECTION ( 'NONE',  ( -1.000000000000000000, 0.000000000000000000, 0.000000000000000000 ) ) ;
#16084=VERTEX_POINT ( 'NONE', #3859 ) ;
#16104=CARTESIAN_POINT ( 'NONE',  ( -0.5677441908128971759, 0.6261827486008704202, 0.07772707057083097504 ) ) ;
#16133=CARTESIAN_POINT ( 'NONE',  ( 0.5309636003393858328, 0.6324615022621647986, -0.5368779841232129701 ) ) ;
#16171=CARTESIAN_POINT ( 'NONE',  ( 0.4898768902087983768, -1.617596456692913393E-16, -0.07874015748031495954 ) ) ;
#16184=CARTESIAN_POINT ( 'NONE',  ( -0.4280150452258433269, -0.6326300546481929965, -0.3109213582405842557 ) ) ;
#16189=ORIENTED_EDGE ( 'NONE', *, *, #23474, .F. ) ;
#16196=CARTESIAN_POINT ( 'NONE',  ( -0.4223526811679828574, -0.5446405551315159910, -0.4444161484266240802 ) ) ;
#16203=CARTESIAN_POINT ( 'NONE',  ( -0.7432982829791772161, 0.3208553412839740826, 0.1963361843227200976 ) ) ;
#16206=CARTESIAN_POINT ( 'NONE',  ( -0.2490711204941342405, 1.208528701367826752, -0.6047752023237676910 ) ) ;
#16208=CARTESIAN_POINT ( 'NONE',  ( 0.5075887755601056206, 1.024205082384598509, -0.2696197026301838107 ) ) ;
#16258=ORIENTED_EDGE ( 'NONE', *, *, #25744, .F. ) ;
#16262=CARTESIAN_POINT ( 'NONE',  ( 0.3976891862754212137, 1.133679329692560245, -0.4395307839725697274 ) ) ;
#16268=ORIENTED_EDGE ( 'NONE', *, *, #13152, .F. ) ;
#16339=CARTESIAN_POINT ( 'NONE',  ( -0.7246715730664488042, 0.2518900982766236196, 0.2118286996268641809 ) ) ;
#16367=CARTESIAN_POINT ( 'NONE',  ( 0.7871730179869745880, 0.4038169352867496120, 0.1713250154738354125 ) ) ;
#16374=ORIENTED_EDGE ( 'NONE', *, *, #17360, .F. ) ;
#16385=CARTESIAN_POINT ( 'NONE',  ( -0.6100071611449719988, -0.1652942696472855522, 0.2255770376035045044 ) ) ;
#16397=CARTESIAN_POINT ( 'NONE',  ( -0.7874015748031496509, 5.862181872755905604E-06, -1.869015748010449007 ) ) ;
#16424=ORIENTED_EDGE ( 'NONE', *, *, #9138, .T. ) ;
#16440=CARTESIAN_POINT ( 'NONE',  ( 0.6882266799383700562, -0.2663285262597259728, -0.2694682288251842861 ) ) ;
#16443=SURFACE_STYLE_FILL_AREA ( #16576 ) ;
#16457=CARTESIAN_POINT ( 'NONE',  ( -0.4609540795476803621, -0.4491800479312370031, -0.3703714726251385869 ) ) ;
#16460=ORIENTED_EDGE ( 'NONE', *, *, #9380, .T. ) ;
#16468=CARTESIAN_POINT ( 'NONE',  ( -0.3573825339541266133, -0.7156596623968717319, -0.6596724844134214116 ) ) ;
#16469=DIRECTION ( 'NONE',  ( 0.000000000000000000, -0.9984511807834833830, -0.05563487747868002542 ) ) ;
#16480=CARTESIAN_POINT ( 'NONE',  ( -0.3040421205569480145, 1.249037478091203024, -0.7140903627573721435 ) ) ;
#16496=CARTESIAN_POINT ( 'NONE',  ( -0.7874015748031496509, 0.4828108945773819105, 0.1423708153504031348 ) ) ;
#16499=VERTEX_POINT ( 'NONE', #16530 ) ;
#16504=ORIENTED_EDGE ( 'NONE', *, *, #6553, .F. ) ;
#16517=CARTESIAN_POINT ( 'NONE',  ( -0.6062104012196082303, -0.1785888610321556547, 0.2237894313402810087 ) ) ;
#16522=EDGE_LOOP ( 'NONE', ( #27282, #15466, #4210, #17666, #5160, #15514 ) ) ;
#16526=AXIS2_PLACEMENT_3D ( 'NONE', #26197, #15483, #21967 ) ;
#16530=CARTESIAN_POINT ( 'NONE',  ( 0.3976891862754212137, 0.7181140751201200434, -0.6642661073933326943 ) ) ;
#16540=CARTESIAN_POINT ( 'NONE',  ( 0.7872492282968406307, 0.2535447773504393987, -0.2765860549081538555 ) ) ;
#16574=CARTESIAN_POINT ( 'NONE',  ( 0.5890517850735842442, -0.1589264097367456829, -0.07874015748031495954 ) ) ;
#16576=FILL_AREA_STYLE ('',( #16876 ) ) ;
#16594=CARTESIAN_POINT ( 'NONE',  ( -0.5743180011325290657, -0.1838911706806881652, -0.2570840403994941181 ) ) ;
#16602=CARTESIAN_POINT ( 'NONE',  ( -0.2070393714800602414, -0.08522740305600375044, -0.07874015748031495954 ) ) ;
#16605=CARTESIAN_POINT ( 'NONE',  ( -0.5905726622054751074, -0.1477137071932877743, -0.2496838636049826254 ) ) ;
#16614=EDGE_CURVE ( 'NONE', #5599, #26227, #7881, .T. ) ;
#16618=COLOUR_RGB ( '', 0.40784314, 0.44705882, 0.49803922) ;
#16620=CARTESIAN_POINT ( 'NONE',  ( -0.3334645669291338987, 0.8151331854455394765, -1.007197927683596506 ) ) ;
#16672=CARTESIAN_POINT ( 'NONE',  ( -0.6019536057979716359, -0.1934596109017840404, 0.2216182498624969244 ) ) ;
#16710=ORIENTED_EDGE ( 'NONE', *, *, #14034, .F. ) ;
#16712=CARTESIAN_POINT ( 'NONE',  ( 0.3339160553493882300, 1.241955529277656956, -0.7081600496628898123 ) ) ;
#16734=CARTESIAN_POINT ( 'NONE',  ( -0.5439522672647024715, -0.3503951963723378471, 0.02327463819225972577 ) ) ;
#16803=B_SPLINE_SURFACE_WITH_KNOTS ( 'NONE', 3, 3, ( 
 ( #9977, #16480, #5610, #20857 ),
 ( #24659, #27221, #5758, #1506 ),
 ( #12100, #22558, #955, #20719 ),
 ( #18730, #1365, #8015, #16620 ) ),
 .UNSPECIFIED., .F., .F., .F.,
 ( 4, 4 ),
 ( 4, 4 ),
 ( -0.1875000000000000000, 0.5625000000000000000 ),
 ( -0.2617993877991500185, 0.2617993877991500185 ),
 .UNSPECIFIED. ) ;
#16809=DIRECTION ( 'NONE',  ( 1.000000000000000000, 0.000000000000000000, 0.000000000000000000 ) ) ;
#16813=CARTESIAN_POINT ( 'NONE',  ( -0.6023373761219545930, -0.1921201442084726485, 0.2218210095010204053 ) ) ;
#16864=CLOSED_SHELL ( 'NONE', ( #20339, #22513, #26064, #483, #14245, #12915, #11184, #26848, #27434, #7953, #6259, #20317, #10756, #24663, #8773, #7248, #1955, #7797, #3106, #8649, #10942, #7138, #15367, #10526, #18808, #7705, #11802, #1667, #12951 ) ) ;
#16867=ORIENTED_EDGE ( 'NONE', *, *, #19489, .T. ) ;
#16876=FILL_AREA_STYLE_COLOUR ( '', #16618 ) ;
#16887=CARTESIAN_POINT ( 'NONE',  ( -0.6068752646683485130, -0.1116593662105169332, -0.2438664148410240040 ) ) ;
#16900=CARTESIAN_POINT ( 'NONE',  ( -0.5857032253883902584, -0.1585179380598580323, -0.2517153213116811727 ) ) ;
#16903=ORIENTED_EDGE ( 'NONE', *, *, #27839, .T. ) ;
#16905=DIRECTION ( 'NONE',  ( 0.000000000000000000, 1.000000000000000000, 0.000000000000000000 ) ) ;
#16914=CARTESIAN_POINT ( 'NONE',  ( 0.6175000359513720394, 0.5735261876549937465, -0.4659829881745126134 ) ) ;
#16929=VERTEX_POINT ( 'NONE', #5568 ) ;
#16940=AXIS2_PLACEMENT_3D ( 'NONE', #15007, #23624, #13001 ) ;
#16952=CARTESIAN_POINT ( 'NONE',  ( -0.5356467622208501700, -0.4294193594449044471, 0.1625794819182737050 ) ) ;
#17005=CARTESIAN_POINT ( 'NONE',  ( 0.2249706821157846648, -0.9514344361775100012, -0.1680475531490076835 ) ) ;
#17010=DIRECTION ( 'NONE',  ( 0.000000000000000000, 0.000000000000000000, 1.000000000000000000 ) ) ;
#17013=B_SPLINE_CURVE_WITH_KNOTS ( 'NONE', 3,
 ( #11114, #17862, #15101, #19734, #13365, #26089 ),
 .UNSPECIFIED., .F., .F.,
 ( 4, 1, 1, 4 ),
 ( 0.000000000000000000, 0.4285714285714280480, 0.7142857142857139685, 1.000000000000000000 ),
 .UNSPECIFIED. ) ;
#17023=EDGE_LOOP ( 'NONE', ( #6554, #21897, #24404, #23016, #10379, #10082, #27278 ) ) ;
#17024=CARTESIAN_POINT ( 'NONE',  ( -0.6068752646683485130, -0.1762754969233277791, 0.2241499015451751953 ) ) ;
#17033=CARTESIAN_POINT ( 'NONE',  ( -0.1981752911889803626, -0.1315891372465754772, 0.2362204724409455170 ) ) ;
#17037=CARTESIAN_POINT ( 'NONE',  ( -0.6233626497309882053, -0.07482011975815597293, -0.2396529498863955721 ) ) ;
#17049=VECTOR ( 'NONE', #18500, 39.37007874015748143 ) ;
#17079=CARTESIAN_POINT ( 'NONE',  ( 0.4563908000639795848, 0.9448480804523937682, -0.4282964253270322708 ) ) ;
#17086=CARTESIAN_POINT ( 'NONE',  ( -0.6003276630397328395, -0.1991340584959632176, 0.2207559493283942353 ) ) ;
#17098=ORIENTED_EDGE ( 'NONE', *, *, #2158, .F. ) ;
#17118=LINE ( 'NONE', #17389, #288 ) ;
#17158=CARTESIAN_POINT ( 'NONE',  ( -0.5632721120450597807, -0.2893425403402185014, 0.04127604646039393504 ) ) ;
#17173=CARTESIAN_POINT ( 'NONE',  ( -0.6099157123460891006, -0.1048986197189705483, -0.2429871477880080621 ) ) ;
#17176=CARTESIAN_POINT ( 'NONE',  ( 0.3334645669291338987, -0.9395870660861969093, -0.7720950382133976442 ) ) ;
#17186=CARTESIAN_POINT ( 'NONE',  ( 0.7430739993161732393, 0.4449930158387386259, -0.3601246575843464748 ) ) ;
#17202=CARTESIAN_POINT ( 'NONE',  ( 0.3339160553493882300, 0.7867001919223544082, -0.8344257386302499357 ) ) ;
#17265=EDGE_CURVE ( 'NONE', #26289, #7632, #24809, .T. ) ;
#17292=CARTESIAN_POINT ( 'NONE',  ( -0.6370261810203012853, -0.06082699205827991895, 0.07717020748573424904 ) ) ;
#17302=CARTESIAN_POINT ( 'NONE',  ( -0.6722178168900768691, 0.04410929521222984456, -0.07961573540161062668 ) ) ;
#17320=ORIENTED_EDGE ( 'NONE', *, *, #24972, .T. ) ;
#17360=EDGE_CURVE ( 'NONE', #24281, #6591, #12028, .T. ) ;
#17364=CARTESIAN_POINT ( 'NONE',  ( -0.3622090647521423734, -1.108209299994242114, -0.3946014861199982349 ) ) ;
#17389=CARTESIAN_POINT ( 'NONE',  ( 0.3339160553493877859, 5.862181872755905604E-06, -1.869015748010449007 ) ) ;
#17437=CARTESIAN_POINT ( 'NONE',  ( -0.7874015748031496509, 0.3058301319751310920, -0.2956682880063846164 ) ) ;
#17446=VECTOR ( 'NONE', #8824, 39.37007874015748143 ) ;
#17487=CARTESIAN_POINT ( 'NONE',  ( 0.6808530955049936217, 0.7992025625531264943, -0.04107133681405187448 ) ) ;
#17517=CARTESIAN_POINT ( 'NONE',  ( -0.6562077975700374433, -1.365924015748031427E-17, -0.2362204724409449064 ) ) ;
#17528=STYLED_ITEM ( 'NONE', ( #6149 ), #3396 ) ;
#17559=CARTESIAN_POINT ( 'NONE',  ( -0.3334645669291338987, 5.862181872992126152E-06, -1.869015748010449007 ) ) ;
#17577=DIRECTION ( 'NONE',  ( 0.000000000000000000, 0.000000000000000000, 1.000000000000000000 ) ) ;
#17579=CARTESIAN_POINT ( 'NONE',  ( -0.6633461167951516524, 0.01962289458785622040, -0.07887503487148522785 ) ) ;
#17621=AXIS2_PLACEMENT_3D ( 'NONE', #22987, #5754, #23271 ) ;
#17624=CARTESIAN_POINT ( 'NONE',  ( 0.7434810862212987148, 0.6612525179033372780, 0.05419551519301178677 ) ) ;
#17651=LINE ( 'NONE', #6937, #8688 ) ;
#17666=ORIENTED_EDGE ( 'NONE', *, *, #25563, .F. ) ;
#17677=CARTESIAN_POINT ( 'NONE',  ( 0.4895462770358314786, 0.7878044190917184997, -0.4800777499788905778 ) ) ;
#17696=EDGE_CURVE ( 'NONE', #13891, #6621, #22728, .T. ) ;
#17699=VERTEX_POINT ( 'NONE', #20473 ) ;
#17747=CARTESIAN_POINT ( 'NONE',  ( 0.2083728861314909642, 0.5236634780160394076, -0.008584350130356221617 ) ) ;
#17749=CARTESIAN_POINT ( 'NONE',  ( 0.7205383896161363655, 0.7193007239719539925, 0.01696726750475779227 ) ) ;
#17800=LINE ( 'NONE', #15445, #20553 ) ;
#17811=CARTESIAN_POINT ( 'NONE',  ( 0.7430739993161732393, 0.5308305074509503951, -0.2265429684943779665 ) ) ;
#17828=CARTESIAN_POINT ( 'NONE',  ( -0.6208708315385689236, -0.1269810289789476410, 0.2299899736262448757 ) ) ;
#17837=CARTESIAN_POINT ( 'NONE',  ( -0.7874015748031496509, 0.4238173070432976197, -0.003642219101859409287 ) ) ;
#17862=CARTESIAN_POINT ( 'NONE',  ( 0.3334645669291338987, -0.7876517371453680694, -0.8174568431611989316 ) ) ;
#17872=ORIENTED_EDGE ( 'NONE', *, *, #11071, .F. ) ;
#17889=DIRECTION ( 'NONE',  ( 0.000000000000000000, 0.000000000000000000, 1.000000000000000000 ) ) ;
#17897=AXIS2_PLACEMENT_3D ( 'NONE', #20263, #921, #2867 ) ;
#17910=CARTESIAN_POINT ( 'NONE',  ( -0.6300376947287432694, -0.09431800512982742302, 0.2327803123842870359 ) ) ;
#17934=CARTESIAN_POINT ( 'NONE',  ( 0.7872492035923605025, 0.3513616474746652507, 0.02280110086181263637 ) ) ;
#17942=LINE ( 'NONE', #9479, #13915 ) ;
#17950=CARTESIAN_POINT ( 'NONE',  ( 0.05882388396542066050, 0.8433682279986742802, -0.06931269535625812772 ) ) ;
#17995=CARTESIAN_POINT ( 'NONE',  ( -0.3338887748335572225, -0.7960395739734442699, -0.8657810409865404067 ) ) ;
#18000=CARTESIAN_POINT ( 'NONE',  ( -0.6722178168900768691, 0.05837462721528850068, 0.2350617247236460594 ) ) ;
#18011=PLANE ( 'NONE',  #8737 ) ;
#18064=CARTESIAN_POINT ( 'NONE',  ( 0.5309636003393858328, 0.6336838567619331730, -0.5358812336713733027 ) ) ;
#18097=CARTESIAN_POINT ( 'NONE',  ( 0.3339160553493877859, 9.254566434645669797E-06, -2.341456692880161228 ) ) ;
#18116=CARTESIAN_POINT ( 'NONE',  ( -0.3861436020174326966, -0.7598757196877184983, -0.4401329610783228929 ) ) ;
#18128=CARTESIAN_POINT ( 'NONE',  ( -0.2602238532265429005, 0.000000000000000000, 0.07874015748031495954 ) ) ;
#18134=CARTESIAN_POINT ( 'NONE',  ( -0.3338887748335570560, -0.8039705855317598182, -0.9107153245080098491 ) ) ;
#18142=CARTESIAN_POINT ( 'NONE',  ( -0.2490711204941342405, 0.7655264129003995777, -0.7689379837741201484 ) ) ;
#18186=CARTESIAN_POINT ( 'NONE',  ( -0.2602238532265429005, 0.000000000000000000, 0.2362204724409449064 ) ) ;
#18197=CARTESIAN_POINT ( 'NONE',  ( -0.6108456259501230390, -0.1623518946918469374, 0.2259549200537961378 ) ) ;
#18217=CARTESIAN_POINT ( 'NONE',  ( 0.6175000359513720394, 0.9054199137833151001, -0.1265032560721565114 ) ) ;
#18269=FACE_OUTER_BOUND ( 'NONE', #11592, .T. ) ;
#18280=CARTESIAN_POINT ( 'NONE',  ( 0.7874015748031497619, 0.3447235678987860541, 0.02357451147970114971 ) ) ;
#18281=CARTESIAN_POINT ( 'NONE',  ( -0.08294224740493445769, -0.3759928968107512648, 0.2015410452432984389 ) ) ;
#18283=CARTESIAN_POINT ( 'NONE',  ( -0.3361686847406328282, -0.7841026825723664828, -0.8202046661941250205 ) ) ;
#18287=ORIENTED_EDGE ( 'NONE', *, *, #1786, .F. ) ;
#18326=CARTESIAN_POINT ( 'NONE',  ( -0.5072939182192724994, -0.3381818976696540080, -0.3094365891633428789 ) ) ;
#18335=UNCERTAINTY_MEASURE_WITH_UNIT (LENGTH_MEASURE( 1.000000000000000082E-05 ), #27464, 'distance_accuracy_value', 'NONE') ;
#18339=CARTESIAN_POINT ( 'NONE',  ( -0.6098875082770396361, -0.1657139659499494710, 0.2255226463234533685 ) ) ;
#18375=CARTESIAN_POINT ( 'NONE',  ( 0.4895462770359960136, 1.042587244177305195, -0.2949132003431571003 ) ) ;
#18390=EDGE_LOOP ( 'NONE', ( #7679, #24414, #15984 ) ) ;
#18414=CARTESIAN_POINT ( 'NONE',  ( -0.3681444341728476455, -0.9492712497839211894, -0.4325618785000000521 ) ) ;
#18417=EDGE_LOOP ( 'NONE', ( #13145, #2726, #16903, #10478, #8262, #4168, #18827, #22587 ) ) ;
#18484=CARTESIAN_POINT ( 'NONE',  ( -0.6280286859446104764, -0.1014897488084370580, 0.2322205965604635103 ) ) ;
#18500=DIRECTION ( 'NONE',  ( -1.000000000000000000, 0.000000000000000000, 0.000000000000000000 ) ) ;
#18522=CARTESIAN_POINT ( 'NONE',  ( 0.4245040230928834313, 0.7010584879324154306, -0.6327280771288582573 ) ) ;
#18549=ORIENTED_EDGE ( 'NONE', *, *, #16614, .T. ) ;
#18554=CARTESIAN_POINT ( 'NONE',  ( -0.4101012214746874163, -0.7973509628734607446, -0.2476620753154787635 ) ) ;
#18561=B_SPLINE_SURFACE_WITH_KNOTS ( 'NONE', 3, 3, ( 
 ( #2142, #12873, #25928, #21418, #8556, #2055 ),
 ( #119, #17176, #10667, #6720, #19288, #25790 ),
 ( #20888, #23022, #8692, #6646, #6438, #10952 ),
 ( #8825, #10529, #15358, #4456, #23950, #23685 ) ),
 .UNSPECIFIED., .F., .F., .F.,
 ( 4, 4 ),
 ( 4, 1, 1, 4 ),
 ( -0.1429447353023790002, 0.1429447353023790002 ),
 ( -0.2617993877991500185, -0.03739991254273600241, 0.1121997376282070080, 0.2617993877991500185 ),
 .UNSPECIFIED. ) ;
#18580=CARTESIAN_POINT ( 'NONE',  ( -0.7874015748031496509, 0.9829781505553011334, -0.2190361720152886049 ) ) ;
#18584=ORIENTED_EDGE ( 'NONE', *, *, #7364, .T. ) ;
#18618=CARTESIAN_POINT ( 'NONE',  ( -0.3480868068226445344, 0.1863314354528550765, 0.2260787492974006274 ) ) ;
#18625=CARTESIAN_POINT ( 'NONE',  ( -0.5950316419613312924, -0.2176117105159648402, 0.2177171427811122051 ) ) ;
#18679=CARTESIAN_POINT ( 'NONE',  ( 0.4898768902087983768, -1.879168897637795438E-16, 0.07874015748031495954 ) ) ;
#18687=CARTESIAN_POINT ( 'NONE',  ( 0.4895462770359960136, 0.6604130065487362478, -0.5726600247964968027 ) ) ;
#18714=VERTEX_POINT ( 'NONE', #22719 ) ;
#18730=CARTESIAN_POINT ( 'NONE',  ( -0.2490711204941342405, 0.7655264129003995777, -0.7689379837741201484 ) ) ;
#18738=CARTESIAN_POINT ( 'NONE',  ( 0.4898768902087983768, 0.000000000000000000, 0.2362204724409449064 ) ) ;
#18747=CARTESIAN_POINT ( 'NONE',  ( -0.3040421205569480145, 0.7911861580938169825, -0.8381822164908544481 ) ) ;
#18768=DIRECTION ( 'NONE',  ( 1.000000000000000000, 0.000000000000000000, 0.000000000000000000 ) ) ;
#18773=CARTESIAN_POINT ( 'NONE',  ( -0.6020290825756511310, -0.1931961917790488426, 0.2216582221849488499 ) ) ;
#18804=( GEOMETRIC_REPRESENTATION_CONTEXT ( 3 ) GLOBAL_UNCERTAINTY_ASSIGNED_CONTEXT ( ( #20341 ) ) GLOBAL_UNIT_ASSIGNED_CONTEXT ( ( #21616, #8205, #25711 ) ) REPRESENTATION_CONTEXT ( 'NONE', 'WORKASPACE' ) ) ;
#18806=PRODUCT_DEFINITION_SHAPE ( 'NONE', 'NONE',  #19482 ) ;
#18808=ADVANCED_FACE ( 'NONE', ( #6434 ), #1904, .F. ) ;
#18827=ORIENTED_EDGE ( 'NONE', *, *, #3452, .T. ) ;
#18838=CARTESIAN_POINT ( 'NONE',  ( -0.4609540795476803621, -0.7091159375545984522, 0.02443766350357295600 ) ) ;
#18851=CARTESIAN_POINT ( 'NONE',  ( -0.4869030747914831481, -0.3865778435145336145, -0.3331566184376838491 ) ) ;
#18913=CARTESIAN_POINT ( 'NONE',  ( -0.5536325768349827925, -0.3642082843426176497, 0.1838265301724124334 ) ) ;
#18939=LINE ( 'NONE', #22913, #4643 ) ;
#18989=CARTESIAN_POINT ( 'NONE',  ( -0.5935113537020059171, -0.1956639913954956733, 0.06179785775180177826 ) ) ;
#18993=CARTESIAN_POINT ( 'NONE',  ( 0.7871730179869350641, 0.2557924603611196890, -0.2773276354978094771 ) ) ;
#18994=VERTEX_POINT ( 'NONE', #18580 ) ;
#19002=CARTESIAN_POINT ( 'NONE',  ( -0.5390321293728450591, -0.2641768698347569111, -0.2800551229596216496 ) ) ;
#19023=CARTESIAN_POINT ( 'NONE',  ( -0.6995386212070490162, 0.5414171171806005933, -0.4387325693061223664 ) ) ;
#19033=CARTESIAN_POINT ( 'NONE',  ( 0.3976891862754212137, 1.133679329692560911, -0.4395307839725692833 ) ) ;
#19046=B_SPLINE_SURFACE_WITH_KNOTS ( 'NONE', 3, 3, ( 
 ( #14832, #14964, #6469, #19033 ),
 ( #23713, #6063, #25684, #12817 ),
 ( #21449, #20, #4074, #8585 ),
 ( #17202, #2221, #10842, #19456 ) ),
 .UNSPECIFIED., .F., .F., .F.,
 ( 4, 4 ),
 ( 4, 4 ),
 ( 0.000000000000000000, 1.000000000000000000 ),
 ( -1.199999999999999956, 0.000000000000000000 ),
 .UNSPECIFIED. ) ;
#19055=CARTESIAN_POINT ( 'NONE',  ( -0.6027608817597299717, -0.1906417529132624356, 0.2220433626720438591 ) ) ;
#19064=LENGTH_MEASURE_WITH_UNIT ( LENGTH_MEASURE( 0.02539999999999999897 ), #12985 ) ;
#19066=AXIS2_PLACEMENT_3D ( 'NONE', #27880, #8103, #4004 ) ;
#19083=ORIENTED_EDGE ( 'NONE', *, *, #3452, .F. ) ;
#19092=EDGE_LOOP ( 'NONE', ( #26455, #19175, #2345, #4220, #23707, #20385, #5217, #14693, #2343 ) ) ;
#19097=ORIENTED_EDGE ( 'NONE', *, *, #6553, .T. ) ;
#19128=CARTESIAN_POINT ( 'NONE',  ( -0.5355664161054535244, -0.3246709447438385632, -0.1343123395640568873 ) ) ;
#19138=CARTESIAN_POINT ( 'NONE',  ( -0.01202960507629146324, -0.5140881368932568307, 0.1365555443425394977 ) ) ;
#19142=CARTESIAN_POINT ( 'NONE',  ( -0.5981339658092079681, -0.1309848305394583079, -0.2467760297474455855 ) ) ;
#19175=ORIENTED_EDGE ( 'NONE', *, *, #27839, .F. ) ;
#19200=CARTESIAN_POINT ( 'NONE',  ( -0.5350618161473178480, -0.4315538544190011261, 0.1618230966487632372 ) ) ;
#19271=CARTESIAN_POINT ( 'NONE',  ( -0.4769977115679039370, -0.4103508094347110280, -0.3464985434502441120 ) ) ;
#19285=CARTESIAN_POINT ( 'NONE',  ( -0.5930505946656516869, -0.1422258853902071407, -0.2487018284346101948 ) ) ;
#19288=CARTESIAN_POINT ( 'NONE',  ( 0.1532705055535415473, -0.6139925424104980545, -0.2937959843914932923 ) ) ;
#19327=CARTESIAN_POINT ( 'NONE',  ( 0.4898768902087983768, 0.000000000000000000, -0.2362204724409449064 ) ) ;
#19377=FACE_OUTER_BOUND ( 'NONE', #18390, .T. ) ;
#19409=EDGE_CURVE ( 'NONE', #20656, #21760, #10767, .T. ) ;
#19414=CARTESIAN_POINT ( 'NONE',  ( -0.4995226175161708859, -0.3565589576102653480, -0.3180767762144185440 ) ) ;
#19423=CARTESIAN_POINT ( 'NONE',  ( -0.6806799598997224088, 0.06756148199031772328, -0.08096199836402361016 ) ) ;
#19429=CARTESIAN_POINT ( 'NONE',  ( -0.6869867706933208140, 0.6386884284781711996, -0.3000169784712433119 ) ) ;
#19456=CARTESIAN_POINT ( 'NONE',  ( 0.3339160553493882300, 1.241955529277657622, -0.7081600496628897012 ) ) ;
#19482=PRODUCT_DEFINITION ( 'UNKNOWN', '', #12983, #9944 ) ;
#19484=EDGE_CURVE ( 'NONE', #21760, #23475, #341, .T. ) ;
#19489=EDGE_CURVE ( 'NONE', #22369, #16929, #22573, .T. ) ;
#19504=DIRECTION ( 'NONE',  ( 0.000000000000000000, 0.000000000000000000, 1.000000000000000000 ) ) ;
#19554=CARTESIAN_POINT ( 'NONE',  ( -0.6305589872448129629, -0.09245759066824232875, 0.2329406148073893679 ) ) ;
#19569=CARTESIAN_POINT ( 'NONE',  ( -0.6587140840999922142, 0.006880217451793542785, -0.07874015870966023789 ) ) ;
#19619=CARTESIAN_POINT ( 'NONE',  ( 0.4245040230929275626, 0.8362902341299607301, -0.5517326013040156907 ) ) ;
#19623=CARTESIAN_POINT ( 'NONE',  ( 0.6963683772927192761, 0.7698450987802122336, -0.01895869795567349525 ) ) ;
#19628=LINE ( 'NONE', #15659, #10079 ) ;
#19703=CARTESIAN_POINT ( 'NONE',  ( -0.6633461167951516524, 0.01644978644481641730, -0.2363335391394980334 ) ) ;
#19718=LINE ( 'NONE', #15214, #9893 ) ;
#19734=CARTESIAN_POINT ( 'NONE',  ( 0.2249706821157846648, -0.6026734741281122298, -0.4922986699466661009 ) ) ;
#19750=CARTESIAN_POINT ( 'NONE',  ( 0.6209510983512002147, 0.8905375929024810233, -0.1208886179116861054 ) ) ;
#19799=DIRECTION ( 'NONE',  ( 0.000000000000000000, 0.9847781868929990079, -0.1738157720684100072 ) ) ;
#19800=CARTESIAN_POINT ( 'NONE',  ( -0.7874015748031496509, 0.000000000000000000, -1.052618110236220428 ) ) ;
#19824=CARTESIAN_POINT ( 'NONE',  ( -0.6305589872448129629, -0.05856602962723583133, -0.2382980545837602715 ) ) ;
#19838=CARTESIAN_POINT ( 'NONE',  ( -0.6562077975700097987, -8.659590551181102767E-14, 0.07874015748031495954 ) ) ;
#19848=DIRECTION ( 'NONE',  ( 0.000000000000000000, 0.000000000000000000, -1.000000000000000000 ) ) ;
#19852=SHAPE_REPRESENTATION ( 'Barrel Cam', ( #11588 ), #18804 ) ;
#19885=CARTESIAN_POINT ( 'NONE',  ( 0.4898768902087983768, -2.712048031496063190E-16, -0.2362204724409449064 ) ) ;
#19913=CARTESIAN_POINT ( 'NONE',  ( 0.7874015748031496509, 0.000000000000000000, -1.052618110236220428 ) ) ;
#19921=CARTESIAN_POINT ( 'NONE',  ( 0.7874015748031496509, 5.862181872598426086E-06, -1.869015748010449007 ) ) ;
#19932=EDGE_CURVE ( 'NONE', #17699, #26673, #609, .T. ) ;
#19945=CARTESIAN_POINT ( 'NONE',  ( 0.7873253891977465280, 0.3967224475386726956, 0.1736657078145811273 ) ) ;
#19969=DIRECTION ( 'NONE',  ( -1.000000000000000000, 0.000000000000000000, 0.000000000000000000 ) ) ;
#19972=CARTESIAN_POINT ( 'NONE',  ( -0.7121770198535963825, 0.1553695409075332712, -0.09097790435992263169 ) ) ;
#19978=CARTESIAN_POINT ( 'NONE',  ( 0.3339160553493877859, 0.000000000000000000, -1.052618110236220428 ) ) ;
#20017=CARTESIAN_POINT ( 'NONE',  ( 0.7871730179869745880, 0.4038169352867496120, 0.1713250154738354125 ) ) ;
#20081=CARTESIAN_POINT ( 'NONE',  ( 0.7872492035923605025, 0.3024535499017155238, -0.1268920345179428144 ) ) ;
#20100=EDGE_CURVE ( 'NONE', #20178, #18714, #4772, .T. ) ;
#20115=CARTESIAN_POINT ( 'NONE',  ( -0.6869867706933208140, 0.8452458407161751452, -0.05661920376100448155 ) ) ;
#20145=CYLINDRICAL_SURFACE ( 'NONE', #26624, 0.8163976377952756325 ) ;
#20149=CARTESIAN_POINT ( 'NONE',  ( -0.7795729917428700917, 0.4543402377591519992, 0.1538738033641767755 ) ) ;
#20178=VERTEX_POINT ( 'NONE', #11049 ) ;
#20214=ORIENTED_EDGE ( 'NONE', *, *, #21049, .F. ) ;
#20222=CARTESIAN_POINT ( 'NONE',  ( 0.7872492035923605025, 0.2520782646455287379, -0.2810771231238101686 ) ) ;
#20263=CARTESIAN_POINT ( 'NONE',  ( 0.3334645669291338987, 0.000000000000000000, -1.052618110236220428 ) ) ;
#20271=CARTESIAN_POINT ( 'NONE',  ( -0.3861436020174326966, -0.8827507391022204608, -0.3410916819343109974 ) ) ;
#20277=EDGE_CURVE ( 'NONE', #22878, #12620, #22944, .T. ) ;
#20281=CARTESIAN_POINT ( 'NONE',  ( 0.7874015748031496509, 0.3931603432736094361, 0.1747896609116821598 ) ) ;
#20317=ADVANCED_FACE ( 'NONE', ( #22616 ), #1009, .F. ) ;
#20318=ORIENTED_EDGE ( 'NONE', *, *, #7468, .F. ) ;
#20339=ADVANCED_FACE ( 'NONE', ( #15704 ), #20494, .T. ) ;
#20341=UNCERTAINTY_MEASURE_WITH_UNIT (LENGTH_MEASURE( 1.000000000000000082E-05 ), #21616, 'distance_accuracy_value', 'NONE') ;
#20382=CARTESIAN_POINT ( 'NONE',  ( -0.7874015748031496509, 5.862181872755905604E-06, -1.869015748010449007 ) ) ;
#20384=CARTESIAN_POINT ( 'NONE',  ( 0.4895462770359960136, 1.042587244177305195, -0.2949132003431571003 ) ) ;
#20385=ORIENTED_EDGE ( 'NONE', *, *, #21647, .T. ) ;
#20411=CARTESIAN_POINT ( 'NONE',  ( -0.3338887748335570560, -0.8039705855317598182, -0.9107153245080098491 ) ) ;
#20429=ORIENTED_EDGE ( 'NONE', *, *, #24264, .F. ) ;
#20434=CARTESIAN_POINT ( 'NONE',  ( 0.5975837919107103158, 0.9212417737170555121, -0.1512753729487469612 ) ) ;
#20473=CARTESIAN_POINT ( 'NONE',  ( 0.3339160553493882300, 1.241955529277656956, -0.7081600496628898123 ) ) ;
#20494=CYLINDRICAL_SURFACE ( 'NONE', #7140, 0.8163976377952756325 ) ;
#20503=CARTESIAN_POINT ( 'NONE',  ( 0.6175000359513720394, 0.5713135641347860672, -0.4682461283617597170 ) ) ;
#20508=EDGE_CURVE ( 'NONE', #12620, #20178, #23343, .T. ) ;
#20553=VECTOR ( 'NONE', #19799, 39.37007874015748143 ) ;
#20572=CARTESIAN_POINT ( 'NONE',  ( -0.4312654560679679561, -0.5223570883078585414, -0.4252037497070341177 ) ) ;
#20584=CARTESIAN_POINT ( 'NONE',  ( 0.5257397301587535265, 1.004902120442729085, -0.2449955022150021589 ) ) ;
#20626=CARTESIAN_POINT ( 'NONE',  ( -0.6346825714933396201, -0.07770321308519005654, 0.2339371447117805369 ) ) ;
#20633=VERTEX_POINT ( 'NONE', #25994 ) ;
#20644=FACE_OUTER_BOUND ( 'NONE', #22618, .T. ) ;
#20649=CARTESIAN_POINT ( 'NONE',  ( -0.3334645669291338987, 1.286842404713327115, -0.9809137335991812146 ) ) ;
#20656=VERTEX_POINT ( 'NONE', #8891 ) ;
#20694=CARTESIAN_POINT ( 'NONE',  ( -0.3503688343903059166, -0.7354936199756122450, -0.6941598510668859356 ) ) ;
#20704=CARTESIAN_POINT ( 'NONE',  ( -0.7874015748031496509, 0.3058301319751310920, -0.2956682880063846164 ) ) ;
#20707=CARTESIAN_POINT ( 'NONE',  ( -0.3509880991366251535, -0.7344191267098763021, -0.6958448607219711590 ) ) ;
#20713=EDGE_LOOP ( 'NONE', ( #26047, #18287, #3578, #24303, #26029, #16258, #11956 ) ) ;
#20719=CARTESIAN_POINT ( 'NONE',  ( -0.3334645669291338987, 0.9723695918681358741, -0.9984365296554585933 ) ) ;
#20720=CARTESIAN_POINT ( 'NONE',  ( -0.7874015748031496509, 0.000000000000000000, -1.052618110236220428 ) ) ;
#20745=CARTESIAN_POINT ( 'NONE',  ( -0.7874015748031496509, 0.3943205132762559462, -0.07664873632799094894 ) ) ;
#20778=DIRECTION ( 'NONE',  ( 0.000000000000000000, -7.180547322999998243E-06, 0.9999999999742198442 ) ) ;
#20815=CARTESIAN_POINT ( 'NONE',  ( 0.5890517850735842442, -0.1332273157280143838, -0.2362204724409449064 ) ) ;
#20817=SURFACE_SIDE_STYLE ('',( #16443 ) ) ;
#20824=EDGE_CURVE ( 'NONE', #7632, #5599, #7664, .T. ) ;
#20825=VECTOR ( 'NONE', #7933, 39.37007874015748143 ) ;
#20838=B_SPLINE_SURFACE_WITH_KNOTS ( 'NONE', 3, 3, ( 
 ( #1332, #16440, #20815, #27187 ),
 ( #12339, #25053, #16574, #16171 ),
 ( #1462, #5716, #7693, #18679 ),
 ( #1602, #5857, #20960, #27461 ) ),
 .UNSPECIFIED., .F., .F., .F.,
 ( 4, 4 ),
 ( 4, 4 ),
 ( -1.199999999999999956, 0.000000000000000000 ),
 ( -5.261281292110230545, -3.749855894370889953 ),
 .UNSPECIFIED. ) ;
#20839=DIRECTION ( 'NONE',  ( -1.000000000000000000, 0.000000000000000000, 0.000000000000000000 ) ) ;
#20843=CARTESIAN_POINT ( 'NONE',  ( -0.5816775848650642677, -0.1674846703394633762, -0.2535625474260125856 ) ) ;
#20857=CARTESIAN_POINT ( 'NONE',  ( -0.3334645669291338987, 1.286842404713327115, -0.9809137335991812146 ) ) ;
#20859=DIRECTION ( 'NONE',  ( 0.000000000000000000, 0.000000000000000000, -1.000000000000000000 ) ) ;
#20868=CARTESIAN_POINT ( 'NONE',  ( 0.7378141273707626846, -0.5132596510569377157, 0.1342805930655029401 ) ) ;
#20888=CARTESIAN_POINT ( 'NONE',  ( 0.3334645669291338987, -1.114423376110021513, -0.8575999861807854785 ) ) ;
#20905=CARTESIAN_POINT ( 'NONE',  ( -0.4703564121420970578, -0.6731208498009066954, 0.04710847534168485784 ) ) ;
#20932=ORIENTED_EDGE ( 'NONE', *, *, #20100, .T. ) ;
#20960=CARTESIAN_POINT ( 'NONE',  ( 0.5890517850735842442, -0.2103245977542082534, 0.2362204724409449064 ) ) ;
#20975=CARTESIAN_POINT ( 'NONE',  ( -0.5935113537020059171, -0.2228995930351641841, 0.2169198626053897849 ) ) ;
#20986=CARTESIAN_POINT ( 'NONE',  ( -0.6108855800013244242, -0.1027495160574083549, -0.2427121449866776470 ) ) ;
#21010=CARTESIAN_POINT ( 'NONE',  ( 0.7874015748031496509, 5.862181872755905604E-06, -1.869015748010449007 ) ) ;
#21012=ORIENTED_EDGE ( 'NONE', *, *, #17360, .T. ) ;
#21041=CARTESIAN_POINT ( 'NONE',  ( -0.5639365699154915701, -0.3272902772321842901, 0.1939717402340199737 ) ) ;
#21043=LINE ( 'NONE', #3658, #2018 ) ;
#21049=EDGE_CURVE ( 'NONE', #20633, #26083, #9400, .T. ) ;
#21062=DIRECTION ( 'NONE',  ( 0.000000000000000000, -7.180547322999998243E-06, 0.9999999999742198442 ) ) ;
#21072=EDGE_LOOP ( 'NONE', ( #9965, #6424, #9313, #10776, #16374, #5520, #14049 ) ) ;
#21115=CARTESIAN_POINT ( 'NONE',  ( -0.5546128944410685380, -0.3166022791122425906, 0.03369876051672000133 ) ) ;
#21129=CARTESIAN_POINT ( 'NONE',  ( -0.6087844546985001770, -0.1074051126585219840, -0.2433141525755926904 ) ) ;
#21139=VECTOR ( 'NONE', #15041, 39.37007874015748143 ) ;
#21143=CARTESIAN_POINT ( 'NONE',  ( 0.4895462770359960136, 0.6604130065487362478, -0.5726600247964968027 ) ) ;
#21189=CARTESIAN_POINT ( 'NONE',  ( -0.4354858238158328398, -0.8080706055940760635, -0.04854564796270125632 ) ) ;
#21261=CARTESIAN_POINT ( 'NONE',  ( -0.4769977115679039370, -0.5686613684786834266, -0.07408240853524410141 ) ) ;
#21272=CARTESIAN_POINT ( 'NONE',  ( 0.05001895696127157259, -0.6334106509489122461, 0.07751973113670669602 ) ) ;
#21276=CARTESIAN_POINT ( 'NONE',  ( -0.6259202480181347283, -0.06905013740392607069, -0.2391457790526826388 ) ) ;
#21282=EDGE_CURVE ( 'NONE', #15456, #26345, #9647, .T. ) ;
#21296=CARTESIAN_POINT ( 'NONE',  ( -0.3480868068226445344, 0.1180291665653972477, -0.2426446119172513127 ) ) ;
#21311=AXIS2_PLACEMENT_3D ( 'NONE', #25093, #8156, #23132 ) ;
#21333=CARTESIAN_POINT ( 'NONE',  ( -0.4622328580205838366, -0.7042455557661343457, 0.02741266141520956948 ) ) ;
#21364=CARTESIAN_POINT ( 'NONE',  ( -0.8725268807032540153, 0.000000000000000000, -1.052618110236220428 ) ) ;
#21387=SURFACE_STYLE_USAGE ( .BOTH. , #20817 ) ;
#21398=CARTESIAN_POINT ( 'NONE',  ( -0.5172021183779732523, -0.3148976862790665576, -0.2992753242159311156 ) ) ;
#21412=CARTESIAN_POINT ( 'NONE',  ( -0.5513845672049195734, -0.2358478765533125465, -0.2710066445262201973 ) ) ;
#21418=CARTESIAN_POINT ( 'NONE',  ( 0.2249706821157846648, -0.6026734741281122298, -0.4922986699466661009 ) ) ;
#21449=CARTESIAN_POINT ( 'NONE',  ( 0.3339160553493882300, 0.7695422168913326200, -0.7725620623222638761 ) ) ;
#21452=ORIENTED_EDGE ( 'NONE', *, *, #6493, .F. ) ;
#21461=CARTESIAN_POINT ( 'NONE',  ( -0.03794311743615354227, 0.6358669483114146592, -0.5146366652944387443 ) ) ;
#21473=CARTESIAN_POINT ( 'NONE',  ( -0.3334645669291338987, 0.8151331854455394765, -1.007197927683596506 ) ) ;
#21507=EDGE_CURVE ( 'NONE', #16084, #26083, #12588, .T. ) ;
#21527=CARTESIAN_POINT ( 'NONE',  ( 0.1120675189988346587, -0.7410715175625038897, 0.001857066358701141805 ) ) ;
#21535=CARTESIAN_POINT ( 'NONE',  ( -0.5632721120450597807, -0.2490672660460055143, -0.1109894576568373897 ) ) ;
#21544=CARTESIAN_POINT ( 'NONE',  ( -0.6722178168900768691, 0.03697663028270673641, -0.2369544657523791342 ) ) ;
#21616=( CONVERSION_BASED_UNIT ( 'INCH', #19064 ) LENGTH_UNIT ( ) NAMED_UNIT ( #10878 ) ) ;
#21647=EDGE_CURVE ( 'NONE', #13891, #1203, #5006, .T. ) ;
#21677=CARTESIAN_POINT ( 'NONE',  ( -0.6262477747318130339, -0.06831769653862618252, -0.2390583512122653465 ) ) ;
#21743=CARTESIAN_POINT ( 'NONE',  ( -0.3615656011995883046, -1.111062966736172219, -0.3994379734395031578 ) ) ;
#21760=VERTEX_POINT ( 'NONE', #10691 ) ;
#21780=CIRCLE ( 'NONE', #9572, 1.288838582677165556 ) ;
#21785=DIRECTION ( 'NONE',  ( 0.000000000000000000, 0.000000000000000000, -1.000000000000000000 ) ) ;
#21798=VECTOR ( 'NONE', #10462, 39.37007874015748143 ) ;
#21811=CARTESIAN_POINT ( 'NONE',  ( -0.6505662911506299162, -0.02047472615278346855, 0.2361156911274059078 ) ) ;
#21823=CARTESIAN_POINT ( 'NONE',  ( -0.6806799598997224088, 0.07848646696189429117, 0.07615904174712244401 ) ) ;
#21897=ORIENTED_EDGE ( 'NONE', *, *, #4995, .T. ) ;
#21908=APPLICATION_CONTEXT ( 'automotive_design' ) ;
#21939=DIRECTION ( 'NONE',  ( -1.000000000000000000, 0.000000000000000000, 0.000000000000000000 ) ) ;
#21940=CARTESIAN_POINT ( 'NONE',  ( 0.3339160553493882300, 1.241955529277656956, -0.7081600496628898123 ) ) ;
#21967=DIRECTION ( 'NONE',  ( 0.000000000000000000, 1.000000000000000000, 0.000000000000000000 ) ) ;
#21981=PRODUCT_CONTEXT ( 'NONE', #614, 'mechanical' ) ;
#22015=CARTESIAN_POINT ( 'NONE',  ( -0.3631207844635358506, -1.104178130233240296, -0.3878391952755386729 ) ) ;
#22020=AXIS2_PLACEMENT_3D ( 'NONE', #23903, #15789, #8770 ) ;
#22050=VERTEX_POINT ( 'NONE', #18993 ) ;
#22062=CARTESIAN_POINT ( 'NONE',  ( 0.7873253891977465280, 0.3482478513048458124, 0.02382806990687684479 ) ) ;
#22082=CARTESIAN_POINT ( 'NONE',  ( 0.4563908000639787521, 1.076366897322332816, -0.3413933471944003428 ) ) ;
#22087=FACE_OUTER_BOUND ( 'NONE', #8106, .T. ) ;
#22090=CARTESIAN_POINT ( 'NONE',  ( -0.6633461167951516524, 0.02596910924942653909, 0.2360419752028775631 ) ) ;
#22121=CARTESIAN_POINT ( 'NONE',  ( -0.7874015748031496509, 0.6226544199590670070, -0.5245967315940827103 ) ) ;
#22143=DIRECTION ( 'NONE',  ( 1.000000000000000000, 0.000000000000000000, 0.000000000000000000 ) ) ;
#22174=CYLINDRICAL_SURFACE ( 'NONE', #11833, 0.4226968503937005295 ) ;
#22199=CARTESIAN_POINT ( 'NONE',  ( 0.7874015748031325534, 0.2970927457007063732, -0.1251225998731516909 ) ) ;
#22217=CARTESIAN_POINT ( 'NONE',  ( -0.6165893942483189338, -0.1421421316221962716, 0.2283979491189897792 ) ) ;
#22224=CARTESIAN_POINT ( 'NONE',  ( 0.3339160553493882300, 0.7867001919223544082, -0.8344257386302499357 ) ) ;
#22236=CARTESIAN_POINT ( 'NONE',  ( -0.2602238532265429005, 0.000000000000000000, 0.07874015748031495954 ) ) ;
#22272=CARTESIAN_POINT ( 'NONE',  ( -0.03794311743615354227, 0.8811800718601279225, -0.3070871000585283506 ) ) ;
#22279=DIRECTION ( 'NONE',  ( 0.000000000000000000, 1.000000000000000000, 0.000000000000000000 ) ) ;
#22280=EDGE_CURVE ( 'NONE', #4466, #26673, #846, .T. ) ;
#22306=DIRECTION ( 'NONE',  ( 0.000000000000000000, 0.000000000000000000, 1.000000000000000000 ) ) ;
#22340=CARTESIAN_POINT ( 'NONE',  ( 0.7872492035923605025, 0.4002696914127111261, 0.1724953616442082838 ) ) ;
#22360=CARTESIAN_POINT ( 'NONE',  ( -0.002755116926490333833, 0.9391221323908144347, -0.1603125978787048322 ) ) ;
#22369=VERTEX_POINT ( 'NONE', #4244 ) ;
#22389=CARTESIAN_POINT ( 'NONE',  ( -0.6587140841000099778, 0.005767656754076102253, -0.2362204724409449064 ) ) ;
#22392=CARTESIAN_POINT ( 'NONE',  ( -0.3338887748335567229, -0.9504046458032088251, -0.8343382454507303203 ) ) ;
#22481=CIRCLE ( 'NONE', #22020, 0.8163976377952757435 ) ;
#22484=CARTESIAN_POINT ( 'NONE',  ( 0.7872492035923605025, 0.2525673450849091339, -0.2795801805159861542 ) ) ;
#22503=CARTESIAN_POINT ( 'NONE',  ( -0.2490711204941346568, 1.208528701367826752, -0.6047752023237676910 ) ) ;
#22513=ADVANCED_FACE ( 'NONE', ( #8752 ), #4515, .T. ) ;
#22535=CARTESIAN_POINT ( 'NONE',  ( -0.3861436020174326966, -0.6370004219456083527, -0.5391745765651102529 ) ) ;
#22542=ORIENTED_EDGE ( 'NONE', *, *, #20277, .T. ) ;
#22555=CARTESIAN_POINT ( 'NONE',  ( -0.1786951194748074845, 0.8740064756424290593, -0.6084677936387519193 ) ) ;
#22558=CARTESIAN_POINT ( 'NONE',  ( -0.3040421205569480145, 0.9438032647596121816, -0.7968182652463602356 ) ) ;
#22573=B_SPLINE_CURVE_WITH_KNOTS ( 'NONE', 3,
 ( #20704, #27068, #11520, #7283 ),
 .UNSPECIFIED., .F., .F.,
 ( 4, 4 ),
 ( -1.199999999999999956, -0.5999999999999999778 ),
 .UNSPECIFIED. ) ;
#22583=ORIENTED_EDGE ( 'NONE', *, *, #14827, .T. ) ;
#22587=ORIENTED_EDGE ( 'NONE', *, *, #13152, .T. ) ;
#22612=EDGE_CURVE ( 'NONE', #16929, #8378, #25765, .T. ) ;
#22616=FACE_OUTER_BOUND ( 'NONE', #7083, .T. ) ;
#22618=EDGE_LOOP ( 'NONE', ( #357, #11551, #24378, #17320, #23253, #1821, #10808, #16268, #12821, #1897, #9856 ) ) ;
#22623=CARTESIAN_POINT ( 'NONE',  ( 0.7845931698711713365, 0.3299597629270051846, -0.3067722674759077450 ) ) ;
#22640=LINE ( 'NONE', #18375, #10161 ) ;
#22673=CARTESIAN_POINT ( 'NONE',  ( -0.4280150452258433269, -0.7349289522583307699, -0.1909859530666125904 ) ) ;
#22680=VERTEX_POINT ( 'NONE', #2924 ) ;
#22682=CARTESIAN_POINT ( 'NONE',  ( -0.08294224740493445769, -0.2841094280683381657, -0.1049447807868563037 ) ) ;
#22719=CARTESIAN_POINT ( 'NONE',  ( -0.7874015748031496509, -3.035194737559055338E-06, -1.475314960619023674 ) ) ;
#22728=LINE ( 'NONE', #13986, #824 ) ;
#22732=ORIENTED_EDGE ( 'NONE', *, *, #24700, .T. ) ;
#22748=VERTEX_POINT ( 'NONE', #3344 ) ;
#22819=CARTESIAN_POINT ( 'NONE',  ( -0.3376790527244098450, -0.9256661064038090858, -0.7381404050695216101 ) ) ;
#22829=CARTESIAN_POINT ( 'NONE',  ( 0.7874015748031151229, 0.2490421840548274757, -0.2751330019808225780 ) ) ;
#22830=FACE_OUTER_BOUND ( 'NONE', #13793, .T. ) ;
#22831=ORIENTED_EDGE ( 'NONE', *, *, #14612, .F. ) ;
#22855=LINE ( 'NONE', #1514, #13960 ) ;
#22878=VERTEX_POINT ( 'NONE', #22121 ) ;
#22892=CARTESIAN_POINT ( 'NONE',  ( -0.5463405388150394115, -0.3905529370662977340, 0.1756562191754173219 ) ) ;
#22913=CARTESIAN_POINT ( 'NONE',  ( 0.3339160553493877859, 9.254566434370079157E-06, -2.341456692880161228 ) ) ;
#22926=CARTESIAN_POINT ( 'NONE',  ( -0.1874921196022230063, 1.163150411085155822, -0.4823193919119450057 ) ) ;
#22931=EDGE_CURVE ( 'NONE', #20633, #26345, #17013, .T. ) ;
#22944=CIRCLE ( 'NONE', #25187, 0.8163976377952757435 ) ;
#22972=CARTESIAN_POINT ( 'NONE',  ( 0.1120675189988346587, -0.4694218845611126678, -0.3846748511993476338 ) ) ;
#22987=CARTESIAN_POINT ( 'NONE',  ( -0.7874015748031496509, 0.000000000000000000, -1.052618110236220428 ) ) ;
#23016=ORIENTED_EDGE ( 'NONE', *, *, #22931, .F. ) ;
#23022=CARTESIAN_POINT ( 'NONE',  ( 0.3334645669291338987, -1.091522395027023640, -0.7267332332655965788 ) ) ;
#23030=CARTESIAN_POINT ( 'NONE',  ( -0.3334645669291338987, 0.000000000000000000, -1.052618110236220428 ) ) ;
#23032=CARTESIAN_POINT ( 'NONE',  ( -0.4468450976383792628, -0.7637389252159438868, -0.01428724896956997704 ) ) ;
#23037=EDGE_CURVE ( 'NONE', #8378, #26227, #13940, .T. ) ;
#23091=( NAMED_UNIT ( * ) SI_UNIT ( $, .STERADIAN. ) SOLID_ANGLE_UNIT ( ) ) ;
#23105=CARTESIAN_POINT ( 'NONE',  ( -0.5833277509429386498, -0.2585366369247649732, 0.2102047045095200573 ) ) ;
#23113=PRODUCT ( 'Barrel Cam', 'Barrel Cam', '', ( #21981 ) ) ;
#23114=CARTESIAN_POINT ( 'NONE',  ( -0.08294224740493465198, -0.3300511624395449095, 0.04829813222822094965 ) ) ;
#23118=CARTESIAN_POINT ( 'NONE',  ( -0.5336559655304955463, -0.2766137621800717206, -0.2845086883298418856 ) ) ;
#23132=DIRECTION ( 'NONE',  ( 0.000000000000000000, 7.180547322999998243E-06, -0.9999999999742198442 ) ) ;
#23176=CARTESIAN_POINT ( 'NONE',  ( -0.5756876931373007267, -0.2855297575254043818, 0.2042278449590817502 ) ) ;
#23228=AXIS2_PLACEMENT_3D ( 'NONE', #13256, #25983, #8878 ) ;
#23250=CARTESIAN_POINT ( 'NONE',  ( -0.5172021183779732523, -0.3756403699547334885, -0.1539580800082084311 ) ) ;
#23253=ORIENTED_EDGE ( 'NONE', *, *, #22280, .T. ) ;
#23271=DIRECTION ( 'NONE',  ( 0.000000000000000000, -7.180547322999999937E-06, -0.9999999999742198442 ) ) ;
#23279=DIRECTION ( 'NONE',  ( 1.000000000000000000, 0.000000000000000000, 0.000000000000000000 ) ) ;
#23328=CARTESIAN_POINT ( 'NONE',  ( -0.5719614286040570761, -0.2987169063169233807, 0.2011802169574927746 ) ) ;
#23335=CARTESIAN_POINT ( 'NONE',  ( -0.2602238532265429005, 0.000000000000000000, -0.2362204724409449064 ) ) ;
#23341=CARTESIAN_POINT ( 'NONE',  ( -0.7874015748031496509, -1.322410629921259858E-32, -0.6299212598425196763 ) ) ;
#23343=LINE ( 'NONE', #16397, #23866 ) ;
#23394=CARTESIAN_POINT ( 'NONE',  ( -0.5252801253069795395, -0.4673450799357756202, 0.1486916858744336545 ) ) ;
#23402=B_SPLINE_CURVE_WITH_KNOTS ( 'NONE', 3,
 ( #13918, #22389, #27056, #26475, #7706, #24364, #13626, #24493, #3010, #11648, #5445, #927, #14058 ),
 .UNSPECIFIED., .F., .F.,
 ( 4, 1, 1, 1, 1, 1, 1, 1, 1, 1, 4 ),
 ( 0.3833360769390280476, 0.3893635454205919832, 0.3944867497131970269, 0.4047331582984080023, 0.4098563625910129904, 0.4201027711762239658, 0.4252259754688289539, 0.4405955883466449730, 0.4508419969318550047, 0.4713348141022760118, 0.4911627496483090272 ),
 .UNSPECIFIED. ) ;
#23409=CARTESIAN_POINT ( 'NONE',  ( -0.6254176984700635655, -0.07018457039985938339, -0.2392426808639660785 ) ) ;
#23467=CARTESIAN_POINT ( 'NONE',  ( -0.5144115741929539132, -0.5069565267453091106, 0.1348810065547058623 ) ) ;
#23468=LINE ( 'NONE', #14852, #7172 ) ;
#23474=EDGE_CURVE ( 'NONE', #18994, #22878, #24562, .T. ) ;
#23475=VERTEX_POINT ( 'NONE', #26406 ) ;
#23512=PLANE ( 'NONE',  #19066 ) ;
#23528=B_SPLINE_CURVE_WITH_KNOTS ( 'NONE', 3,
 ( #12645, #21272, #19138, #27770, #17033, #8411 ),
 .UNSPECIFIED., .F., .F.,
 ( 4, 2, 4 ),
 ( 0.000000000000000000, 0.5000000000000000000, 1.000000000000000000 ),
 .UNSPECIFIED. ) ;
#23532=CARTESIAN_POINT ( 'NONE',  ( -0.4769977115679039370, -0.6478166167414666221, 0.06212561209344763524 ) ) ;
#23546=CARTESIAN_POINT ( 'NONE',  ( -0.6222485084499363994, -0.07732954745974893185, -0.2398894390934003529 ) ) ;
#23552=FACE_OUTER_BOUND ( 'NONE', #24008, .T. ) ;
#23567=CARTESIAN_POINT ( 'NONE',  ( -0.3041553300245939950, 0.05901566860999998831, -0.2362204724409447953 ) ) ;
#23595=B_SPLINE_SURFACE_WITH_KNOTS ( 'NONE', 3, 3, ( 
 ( #19885, #7030, #15915, #2765, #7296, #18142 ),
 ( #26786, #537, #16063, #5170, #22555, #15783 ),
 ( #9128, #24522, #17747, #22272, #26369, #5466 ),
 ( #9694, #3037, #11533, #7579, #11671, #16206 ) ),
 .UNSPECIFIED., .F., .F., .F.,
 ( 4, 4 ),
 ( 4, 1, 1, 4 ),
 ( -1.199999999999999956, 0.000000000000000000 ),
 ( -3.749855894370895282, -2.141060511069079908, -1.068530255534539952, 0.004000000000000000083 ),
 .UNSPECIFIED. ) ;
#23610=B_SPLINE_CURVE_WITH_KNOTS ( 'NONE', 3,
 ( #5537, #16540, #14161, #12457 ),
 .UNSPECIFIED., .F., .F.,
 ( 4, 4 ),
 ( 0.000000000000000000, 0.0001798248967499302582 ),
 .UNSPECIFIED. ) ;
#23624=DIRECTION ( 'NONE',  ( -1.000000000000000000, 0.000000000000000000, 0.000000000000000000 ) ) ;
#23636=CARTESIAN_POINT ( 'NONE',  ( -0.7874015748031496509, -3.035194737716535704E-06, -1.475314960619023674 ) ) ;
#23662=VECTOR ( 'NONE', #11050, 39.37007874015748143 ) ;
#23667=AXIS2_PLACEMENT_3D ( 'NONE', #21364, #75, #2275 ) ;
#23669=CARTESIAN_POINT ( 'NONE',  ( -0.5546128944410685380, -0.3606719828935669447, 0.1849095013362464512 ) ) ;
#23670=CARTESIAN_POINT ( 'NONE',  ( -0.7874015748031496509, 5.862181872598426086E-06, -1.869015748010449007 ) ) ;
#23678=CARTESIAN_POINT ( 'NONE',  ( -0.7246715730664488042, 0.1903343190505137617, -0.09717118172266910048 ) ) ;
#23685=CARTESIAN_POINT ( 'NONE',  ( 0.1120675189988346587, -0.7410715175625038897, 0.001857066358701496122 ) ) ;
#23698=ORIENTED_EDGE ( 'NONE', *, *, #8536, .T. ) ;
#23699=ORIENTED_EDGE ( 'NONE', *, *, #8559, .F. ) ;
#23707=ORIENTED_EDGE ( 'NONE', *, *, #9655, .T. ) ;
#23713=CARTESIAN_POINT ( 'NONE',  ( 0.3561571326799479742, 0.7445305536541476643, -0.7131136604161752990 ) ) ;
#23732=CARTESIAN_POINT ( 'NONE',  ( -0.4031801809406276860, -0.9361362132892122601, -0.1635458728543118245 ) ) ;
#23801=B_SPLINE_CURVE_WITH_KNOTS ( 'NONE', 3,
 ( #22503, #22926, #754, #22360, #17950, #11905, #26585, #2984, #24893, #5113 ),
 .UNSPECIFIED., .F., .F.,
 ( 4, 2, 2, 2, 4 ),
 ( 0.000000000000000000, 0.2500000000000000000, 0.5000000000000000000, 0.7500000000000000000, 1.000000000000000000 ),
 .UNSPECIFIED. ) ;
#23810=CARTESIAN_POINT ( 'NONE',  ( -0.6996199877990079141, 0.1008405537593297374, -0.2423665665178251771 ) ) ;
#23817=CARTESIAN_POINT ( 'NONE',  ( -0.3338887748335570560, -1.269220122646561144, -0.8285976369166339062 ) ) ;
#23819=CARTESIAN_POINT ( 'NONE',  ( 0.7874015748031496509, 0.000000000000000000, -1.052618110236220428 ) ) ;
#23866=VECTOR ( 'NONE', #20778, 39.37007874015748143 ) ;
#23867=CARTESIAN_POINT ( 'NONE',  ( 0.7673390720865624903, 0.5739376981955128798, 0.1014356048888053474 ) ) ;
#23903=CARTESIAN_POINT ( 'NONE',  ( 0.7874015748031496509, 0.000000000000000000, -1.052618110236220428 ) ) ;
#23904=EDGE_LOOP ( 'NONE', ( #20429, #16460, #27694, #1476 ) ) ;
#23944=CARTESIAN_POINT ( 'NONE',  ( -0.7795729917428700917, 0.2877957735339043421, -0.2883818734248744242 ) ) ;
#23950=CARTESIAN_POINT ( 'NONE',  ( 0.1532705055535415473, -0.8125630895486949390, -0.04838628589907047889 ) ) ;
#23972=DIRECTION ( 'NONE',  ( 0.000000000000000000, 0.9984511807834832720, 0.05563487747868100380 ) ) ;
#23975=ORIENTED_EDGE ( 'NONE', *, *, #1435, .T. ) ;
#23980=ORIENTED_EDGE ( 'NONE', *, *, #10164, .T. ) ;
#23986=CARTESIAN_POINT ( 'NONE',  ( 0.4895462770359960136, 0.6604130065487362478, -0.5726600247964968027 ) ) ;
#23989=CARTESIAN_POINT ( 'NONE',  ( 0.6058062761461652235, 0.9107023032972123566, -0.1406092616970065767 ) ) ;
#23990=EDGE_CURVE ( 'NONE', #5887, #3730, #4816, .T. ) ;
#24008=EDGE_LOOP ( 'NONE', ( #13563, #11087, #14354, #16031 ) ) ;
#24041=ORIENTED_EDGE ( 'NONE', *, *, #11071, .T. ) ;
#24047=CARTESIAN_POINT ( 'NONE',  ( 0.7874015748031325534, 0.3931752036646342097, 0.1748360539849539708 ) ) ;
#24058=ORIENTED_EDGE ( 'NONE', *, *, #21282, .F. ) ;
#24066=CARTESIAN_POINT ( 'NONE',  ( -0.6434710025615986151, -0.03484970772117712556, -0.07928083200629056082 ) ) ;
#24075=CARTESIAN_POINT ( 'NONE',  ( -0.6806799598997224088, 0.08941145402117105234, 0.2332800728132976564 ) ) ;
#24093=AXIS2_PLACEMENT_3D ( 'NONE', #26721, #27166, #7668 ) ;
#24118=EDGE_LOOP ( 'NONE', ( #12145, #1982, #10562, #22583, #15509, #1059, #2491, #21012 ) ) ;
#24189=CARTESIAN_POINT ( 'NONE',  ( 0.4895462770358314786, 0.6578651782979850760, -0.5745116702929976560 ) ) ;
#24204=CARTESIAN_POINT ( 'NONE',  ( -0.6262477747318130339, -0.08149594654892677870, -0.08212545458858977465 ) ) ;
#24207=CARTESIAN_POINT ( 'NONE',  ( 0.3976891862754212137, 1.133679329692560245, -0.4395307839725697274 ) ) ;
#24233=CIRCLE ( 'NONE', #17897, 1.288838582677166222 ) ;
#24255=CARTESIAN_POINT ( 'NONE',  ( 0.6939626785200878611, 0.7744396987992381298, -0.02240038148060783177 ) ) ;
#24264=EDGE_CURVE ( 'NONE', #6360, #20178, #8784, .T. ) ;
#24281=VERTEX_POINT ( 'NONE', #2012 ) ;
#24303=ORIENTED_EDGE ( 'NONE', *, *, #25563, .T. ) ;
#24312=ORIENTED_EDGE ( 'NONE', *, *, #27371, .T. ) ;
#24315=CARTESIAN_POINT ( 'NONE',  ( 0.7872492035923605025, 0.2535455059636700370, -0.2765862953003382363 ) ) ;
#24335=CARTESIAN_POINT ( 'NONE',  ( -0.6544535166833030937, -0.006373303606307913032, 0.2362204724409449064 ) ) ;
#24351=DIRECTION ( 'NONE',  ( 0.000000000000000000, 7.180547322999999937E-06, -0.9999999999742198442 ) ) ;
#24360=VERTEX_POINT ( 'NONE', #18097 ) ;
#24364=CARTESIAN_POINT ( 'NONE',  ( -0.6912180915490531152, 0.08120084520073209133, -0.2401638807511342344 ) ) ;
#24375=CARTESIAN_POINT ( 'NONE',  ( 0.7874015748031496509, 0.3326143029362100823, -0.01422925309762631055 ) ) ;
#24378=ORIENTED_EDGE ( 'NONE', *, *, #19409, .F. ) ;
#24389=CARTESIAN_POINT ( 'NONE',  ( -0.8725268807032540153, 0.000000000000000000, -1.052618110236220428 ) ) ;
#24390=CARTESIAN_POINT ( 'NONE',  ( 0.7608910173126012255, 0.6007740188332617581, 0.08763475256689905180 ) ) ;
#24395=CARTESIAN_POINT ( 'NONE',  ( 0.7874015748031496509, -0.3839064563524838825, -0.3321176343386787466 ) ) ;
#24404=ORIENTED_EDGE ( 'NONE', *, *, #21282, .T. ) ;
#24414=ORIENTED_EDGE ( 'NONE', *, *, #17696, .T. ) ;
#24444=CARTESIAN_POINT ( 'NONE',  ( 0.7430739993161732393, 0.4449930158387386259, -0.3601246575843464748 ) ) ;
#24493=CARTESIAN_POINT ( 'NONE',  ( -0.7121770198535963825, 0.1302456093167436990, -0.2464793285356193242 ) ) ;
#24496=CARTESIAN_POINT ( 'NONE',  ( -0.3503688343903059166, -0.8773679034442795066, -0.6250144544381456280 ) ) ;
#24511=CARTESIAN_POINT ( 'NONE',  ( -0.3693533223127509202, -0.6818538191143146410, -0.6013702642917986285 ) ) ;
#24522=CARTESIAN_POINT ( 'NONE',  ( 0.3843128886798078958, 0.1965195625994889950, 0.07874015748031495954 ) ) ;
#24562=LINE ( 'NONE', #9736, #5106 ) ;
#24570=CARTESIAN_POINT ( 'NONE',  ( -0.6385905051800526699, -0.06366962376380753963, 0.2346802187740419654 ) ) ;
#24590=CARTESIAN_POINT ( 'NONE',  ( 0.7430739993161732393, 0.4441346409226165082, -0.3614604744752461518 ) ) ;
#24591=EDGE_CURVE ( 'NONE', #6591, #26289, #11706, .T. ) ;
#24628=ORIENTED_EDGE ( 'NONE', *, *, #5878, .T. ) ;
#24636=CARTESIAN_POINT ( 'NONE',  ( -0.3338887748335567229, -0.7967198305134626235, -0.8696351319825925685 ) ) ;
#24641=VERTEX_POINT ( 'NONE', #72 ) ;
#24655=CARTESIAN_POINT ( 'NONE',  ( 0.4898768902087983768, 0.000000000000000000, -0.2362204724409449064 ) ) ;
#24657=CYLINDRICAL_SURFACE ( 'NONE', #9836, 1.288838582677165556 ) ;
#24659=CARTESIAN_POINT ( 'NONE',  ( -0.2490711204941342405, 1.060861271878683176, -0.6594961294738858060 ) ) ;
#24663=ADVANCED_FACE ( 'NONE', ( #11306 ), #18561, .F. ) ;
#24700=EDGE_CURVE ( 'NONE', #26847, #18994, #7126, .T. ) ;
#24705=CARTESIAN_POINT ( 'NONE',  ( -0.6463085202143212804, -0.03588704011884780165, 0.2358541165544890683 ) ) ;
#24732=CARTESIAN_POINT ( 'NONE',  ( 0.5309636003393858328, 0.6300167932626280498, -0.5388714850268924161 ) ) ;
#24788=ORIENTED_EDGE ( 'NONE', *, *, #22931, .T. ) ;
#24796=CARTESIAN_POINT ( 'NONE',  ( -0.4284035790182393888, -0.5294929124318047409, -0.4312010047435373972 ) ) ;
#24797=FACE_OUTER_BOUND ( 'NONE', #14333, .T. ) ;
#24809=CIRCLE ( 'NONE', #12639, 0.8163976377952757435 ) ;
#24825=ADVANCED_BREP_SHAPE_REPRESENTATION ( 'Barrel Cam', ( #3396, #11588 ), #18804 ) ;
#24893=CARTESIAN_POINT ( 'NONE',  ( 0.4282978893168862267, 0.1305933181008684940, 0.2362204724409449896 ) ) ;
#24911=AXIS2_PLACEMENT_3D ( 'NONE', #8986, #2493, #23972 ) ;
#24923=CARTESIAN_POINT ( 'NONE',  ( -0.3338887748335570560, -0.9590537645700274449, -0.8833427619775512385 ) ) ;
#24931=CARTESIAN_POINT ( 'NONE',  ( -0.08294224740493445769, -0.2381676936971315051, -0.2581876938019334600 ) ) ;
#24967=CARTESIAN_POINT ( 'NONE',  ( -0.2490711204941346568, 0.7655264129003995777, -0.7689379837741201484 ) ) ;
#24970=CARTESIAN_POINT ( 'NONE',  ( 0.7872492283035658067, 0.4002685408453414140, 0.1724957412521976319 ) ) ;
#24972=EDGE_CURVE ( 'NONE', #20656, #4466, #3777, .T. ) ;
#25001=VERTEX_POINT ( 'NONE', #14379 ) ;
#25016=ORIENTED_EDGE ( 'NONE', *, *, #27371, .F. ) ;
#25043=VECTOR ( 'NONE', #10600, 39.37007874015748854 ) ;
#25053=CARTESIAN_POINT ( 'NONE',  ( 0.6882266799383700562, -0.3177023890156830954, -0.1184012924741053158 ) ) ;
#25081=CARTESIAN_POINT ( 'NONE',  ( -0.3792810011673199977, -0.6551894325502299887, -0.5632424446553236930 ) ) ;
#25091=CARTESIAN_POINT ( 'NONE',  ( 0.5664712772799370688, 0.9591943317212182629, -0.1917392787441815627 ) ) ;
#25093=CARTESIAN_POINT ( 'NONE',  ( -0.7874015748031496509, 7.558374153346456878E-06, -2.105236220445303008 ) ) ;
#25116=CARTESIAN_POINT ( 'NONE',  ( 0.7874015748031496509, 0.3931603432736094361, 0.1747896609116821598 ) ) ;
#25123=ORIENTED_EDGE ( 'NONE', *, *, #7556, .T. ) ;
#25139=CARTESIAN_POINT ( 'NONE',  ( -0.5677563751001175607, -0.3136670689571407489, 0.1974823232504523962 ) ) ;
#25187=AXIS2_PLACEMENT_3D ( 'NONE', #19800, #461, #8512 ) ;
#25193=( LENGTH_UNIT ( ) NAMED_UNIT ( * ) SI_UNIT ( $, .METRE. ) ) ;
#25207=CARTESIAN_POINT ( 'NONE',  ( -0.4609540795476803621, -0.5358253718921779374, -0.2387683900552271810 ) ) ;
#25218=CARTESIAN_POINT ( 'NONE',  ( -0.5596283908538459695, -0.2170791976991290062, -0.2655998857763979260 ) ) ;
#25281=CARTESIAN_POINT ( 'NONE',  ( -0.5960173041437835106, -0.2141719054356908680, 0.2183038118118142967 ) ) ;
#25286=VECTOR ( 'NONE', #25370, 39.37007874015748143 ) ;
#25347=CARTESIAN_POINT ( 'NONE',  ( -0.5833277509429386498, -0.1637665899405980618, -0.2526998142065598474 ) ) ;
#25363=CARTESIAN_POINT ( 'NONE',  ( -0.6247226535096832567, -0.07175300650175490957, -0.2393789016825997595 ) ) ;
#25370=DIRECTION ( 'NONE',  ( 0.000000000000000000, 0.000000000000000000, 1.000000000000000000 ) ) ;
#25462=DIRECTION ( 'NONE',  ( 1.000000000000000000, 0.000000000000000000, 0.000000000000000000 ) ) ;
#25494=CARTESIAN_POINT ( 'NONE',  ( -0.2490711204941346568, 1.208528701367826752, -0.6047752023237676910 ) ) ;
#25500=CARTESIAN_POINT ( 'NONE',  ( -0.4995226175161708859, -0.5628959716349646314, 0.1069947647043326677 ) ) ;
#25510=CARTESIAN_POINT ( 'NONE',  ( -0.5943003644086487514, -0.1394605577792424056, -0.2482195849639082796 ) ) ;
#25533=ORIENTED_EDGE ( 'NONE', *, *, #24700, .F. ) ;
#25563=EDGE_CURVE ( 'NONE', #22050, #23475, #23610, .T. ) ;
#25565=DIRECTION ( 'NONE',  ( 0.000000000000000000, -0.9847781868929988969, 0.1738157720684100072 ) ) ;
#25568=CARTESIAN_POINT ( 'NONE',  ( -0.6021528086661247503, -0.1927643575067814197, 0.2217236187994692798 ) ) ;
#25579=CARTESIAN_POINT ( 'NONE',  ( -0.2602238532265429005, 0.000000000000000000, 0.2362204724409449064 ) ) ;
#25636=CARTESIAN_POINT ( 'NONE',  ( -0.6112138326843681302, -0.1020303416107446876, -0.2425959877567988310 ) ) ;
#25648=CARTESIAN_POINT ( 'NONE',  ( -0.6109916490390459032, -0.1025144698334873039, -0.2426823708759043852 ) ) ;
#25684=CARTESIAN_POINT ( 'NONE',  ( 0.3561571326799479742, 1.031746018571391810, -0.5821543563138212862 ) ) ;
#25695=CARTESIAN_POINT ( 'NONE',  ( 0.4563908000639795848, 0.6818102780176417133, -0.6021022548815945230 ) ) ;
#25711=( NAMED_UNIT ( * ) SI_UNIT ( $, .STERADIAN. ) SOLID_ANGLE_UNIT ( ) ) ;
#25733=DIRECTION ( 'NONE',  ( 1.000000000000000000, 0.000000000000000000, 0.000000000000000000 ) ) ;
#25744=EDGE_CURVE ( 'NONE', #22680, #25818, #17118, .T. ) ;
#25765=B_SPLINE_CURVE_WITH_KNOTS ( 'NONE', 3,
 ( #20745, #5632, #5778, #16496 ),
 .UNSPECIFIED., .F., .F.,
 ( 4, 4 ),
 ( -0.5999999999999999778, 0.000000000000000000 ),
 .UNSPECIFIED. ) ;
#25774=CARTESIAN_POINT ( 'NONE',  ( -0.4769977115679039370, -0.4895060576974945010, -0.2102905228215523614 ) ) ;
#25784=CARTESIAN_POINT ( 'NONE',  ( -0.6996199877990079141, 0.1397441489511527524, 0.07022294643182264151 ) ) ;
#25787=CARTESIAN_POINT ( 'NONE',  ( -0.5329937562553743735, -0.2781466909400371335, -0.2850623042816753383 ) ) ;
#25790=CARTESIAN_POINT ( 'NONE',  ( 0.1120675189988346587, -0.5599717622282432972, -0.2558308786799976531 ) ) ;
#25813=EDGE_LOOP ( 'NONE', ( #7443, #22732, #189, #13854 ) ) ;
#25818=VERTEX_POINT ( 'NONE', #19921 ) ;
#25822=FACE_OUTER_BOUND ( 'NONE', #2383, .T. ) ;
#25897=EDGE_CURVE ( 'NONE', #22050, #3563, #5432, .T. ) ;
#25914=CARTESIAN_POINT ( 'NONE',  ( -0.6544535166833030937, -0.005594563712608583567, 0.07874015109845884652 ) ) ;
#25928=CARTESIAN_POINT ( 'NONE',  ( 0.3102399269716953345, -0.7316071111737637578, -0.6652804359117283628 ) ) ;
#25937=EDGE_CURVE ( 'NONE', #1203, #15744, #8490, .T. ) ;
#25947=SHAPE_DEFINITION_REPRESENTATION ( #18806, #19852 ) ;
#25961=ORIENTED_EDGE ( 'NONE', *, *, #2158, .T. ) ;
#25974=CARTESIAN_POINT ( 'NONE',  ( 0.7616545822564796397, 0.5977631770216751406, 0.08921608065419495137 ) ) ;
#25980=DIRECTION ( 'NONE',  ( 0.000000000000000000, -7.180547322999998243E-06, -0.9999999999742198442 ) ) ;
#25983=DIRECTION ( 'NONE',  ( -1.000000000000000000, 0.000000000000000000, 0.000000000000000000 ) ) ;
#25994=CARTESIAN_POINT ( 'NONE',  ( 0.3334645669291338987, -0.8041772776331653771, -0.9118913923173522784 ) ) ;
#26001=AXIS2_PLACEMENT_3D ( 'NONE', #23341, #3967, #53 ) ;
#26029=ORIENTED_EDGE ( 'NONE', *, *, #4798, .F. ) ;
#26044=CARTESIAN_POINT ( 'NONE',  ( -0.6434710025615986151, -0.04048505764336882140, 0.07811204921870905371 ) ) ;
#26047=ORIENTED_EDGE ( 'NONE', *, *, #10426, .T. ) ;
#26064=ADVANCED_FACE ( 'NONE', ( #8765 ), #7974, .T. ) ;
#26066=FACE_OUTER_BOUND ( 'NONE', #27358, .T. ) ;
#26073=EDGE_LOOP ( 'NONE', ( #20932, #13792, #25123, #13823, #16867, #5406, #1915, #7890, #22542, #11560 ) ) ;
#26083=VERTEX_POINT ( 'NONE', #2263 ) ;
#26089=CARTESIAN_POINT ( 'NONE',  ( 0.1120675189988346587, -0.4694218845611126678, -0.3846748511993476338 ) ) ;
#26107=CARTESIAN_POINT ( 'NONE',  ( 0.6427545578076259147, 0.8597063426663432706, -0.09226840441818499883 ) ) ;
#26113=CARTESIAN_POINT ( 'NONE',  ( -0.3617579313041923705, -1.110209215450335796, -0.3979864608631387690 ) ) ;
#26135=CARTESIAN_POINT ( 'NONE',  ( -0.6562077975700453258, 2.612916929133858441E-14, 0.2362204724409449064 ) ) ;
#26184=CARTESIAN_POINT ( 'NONE',  ( -0.6305589872448129629, -0.08116040399610512102, 0.07586106382108366575 ) ) ;
#26192=CARTESIAN_POINT ( 'NONE',  ( -0.7635713814939685262, 0.3957398197978322374, 0.1751423728567907401 ) ) ;
#26197=CARTESIAN_POINT ( 'NONE',  ( -0.3334645669291338987, 1.286842404713327115, -0.9809137335991812146 ) ) ;
#26227=VERTEX_POINT ( 'NONE', #11027 ) ;
#26232=ORIENTED_EDGE ( 'NONE', *, *, #11935, .T. ) ;
#26240=CARTESIAN_POINT ( 'NONE',  ( 0.5994540303786097812, 0.9188646166935047210, -0.1488510697577987707 ) ) ;
#26266=CIRCLE ( 'NONE', #24911, 0.8163976377952752994 ) ;
#26288=CIRCLE ( 'NONE', #9134, 0.4226968503937005295 ) ;
#26289=VERTEX_POINT ( 'NONE', #1131 ) ;
#26297=CARTESIAN_POINT ( 'NONE',  ( 0.7871730179869745880, 0.3051339520022200991, -0.1277767518403383762 ) ) ;
#26328=CARTESIAN_POINT ( 'NONE',  ( -0.6912180915490531152, 0.1125275769341421150, 0.07327540503423307650 ) ) ;
#26330=AXIS2_PLACEMENT_3D ( 'NONE', #23030, #18768, #27686 ) ;
#26345=VERTEX_POINT ( 'NONE', #13760 ) ;
#26369=CARTESIAN_POINT ( 'NONE',  ( -0.1786951194748074845, 1.015337136915029692, -0.5366467491745039453 ) ) ;
#26406=CARTESIAN_POINT ( 'NONE',  ( 0.7874015748031151229, 0.2490421840548274757, -0.2751330019808225780 ) ) ;
#26430=CARTESIAN_POINT ( 'NONE',  ( 0.7845931698711713365, 0.3958995273828118111, -0.1577356437548364521 ) ) ;
#26445=CARTESIAN_POINT ( 'NONE',  ( -0.6262477747318130339, -0.1078524472662568956, 0.2317403423130409423 ) ) ;
#26455=ORIENTED_EDGE ( 'NONE', *, *, #9380, .F. ) ;
#26475=CARTESIAN_POINT ( 'NONE',  ( -0.6722178168900768691, 0.03697663028270673641, -0.2369544657523791342 ) ) ;
#26499=FACE_OUTER_BOUND ( 'NONE', #25813, .T. ) ;
#26524=B_SPLINE_CURVE_WITH_KNOTS ( 'NONE', 3,
 ( #13961, #3481, #12109, #14540, #20868, #1111 ),
 .UNSPECIFIED., .F., .F.,
 ( 4, 2, 4 ),
 ( 0.000000000000000000, 0.5000000000000000000, 1.000000000000000000 ),
 .UNSPECIFIED. ) ;
#26541=EDGE_CURVE ( 'NONE', #527, #7632, #17800, .T. ) ;
#26565=CARTESIAN_POINT ( 'NONE',  ( 0.6175000359513720394, 0.5735261876549937465, -0.4659829881745126134 ) ) ;
#26585=CARTESIAN_POINT ( 'NONE',  ( 0.2435608866411535234, 0.5103801548612577621, 0.1380420446583983662 ) ) ;
#26598=ORIENTED_EDGE ( 'NONE', *, *, #23037, .F. ) ;
#26605=CARTESIAN_POINT ( 'NONE',  ( -0.5112608635011182123, 0.4674461882104614108, 0.01743336272964224679 ) ) ;
#26624=AXIS2_PLACEMENT_3D ( 'NONE', #5311, #944, #13933 ) ;
#26627=CARTESIAN_POINT ( 'NONE',  ( 0.7874015748031496509, 0.3083957742196543061, -0.08983678263938775499 ) ) ;
#26634=CARTESIAN_POINT ( 'NONE',  ( -0.3592839431930354710, -0.7102362189723434582, -0.6500175644856731605 ) ) ;
#26639=CARTESIAN_POINT ( 'NONE',  ( -0.6587140841000099778, 0.009105340598934882554, 0.2362204724409449064 ) ) ;
#26673=VERTEX_POINT ( 'NONE', #16262 ) ;
#26687=CARTESIAN_POINT ( 'NONE',  ( -0.6259985246028595407, -0.1087303358534330439, 0.2316280589008344604 ) ) ;
#26706=CARTESIAN_POINT ( 'NONE',  ( 0.5309636003393858328, 0.6312391477623964242, -0.5378747345750526376 ) ) ;
#26721=CARTESIAN_POINT ( 'NONE',  ( -0.7874015748031496509, 0.000000000000000000, -1.052618110236220428 ) ) ;
#26725=DIRECTION ( 'NONE',  ( 1.000000000000000000, 0.000000000000000000, 0.000000000000000000 ) ) ;
#26772=CARTESIAN_POINT ( 'NONE',  ( 0.7874015748031497619, 0.3568327973771865391, 0.06137828742325460857 ) ) ;
#26773=CARTESIAN_POINT ( 'NONE',  ( 0.1120675189988346587, -0.7410715175625038897, 0.001857066358701141805 ) ) ;
#26783=CARTESIAN_POINT ( 'NONE',  ( -0.7121770198535963825, 0.2056174084053519757, 0.2200249214779901596 ) ) ;
#26786=CARTESIAN_POINT ( 'NONE',  ( 0.4898768902087983768, -3.235192913385827280E-16, -0.07874015748031495954 ) ) ;
#26826=CARTESIAN_POINT ( 'NONE',  ( -0.3041553300245938840, 0.09316743112151353035, 0.2362204724409449896 ) ) ;
#26841=DIRECTION ( 'NONE',  ( 0.000000000000000000, -7.180547322999998243E-06, 0.9999999999742198442 ) ) ;
#26845=DIRECTION ( 'NONE',  ( -1.000000000000000000, 0.000000000000000000, 0.000000000000000000 ) ) ;
#26847=VERTEX_POINT ( 'NONE', #25579 ) ;
#26848=ADVANCED_FACE ( 'NONE', ( #14998 ), #4524, .T. ) ;
#26854=CARTESIAN_POINT ( 'NONE',  ( 0.7873253891977465280, 0.2503290596427080739, -0.2788417078614053857 ) ) ;
#26892=ORIENTED_EDGE ( 'NONE', *, *, #10571, .F. ) ;
#27056=CARTESIAN_POINT ( 'NONE',  ( -0.6633461167951516524, 0.01644978644481641730, -0.2363335391394980334 ) ) ;
#27068=CARTESIAN_POINT ( 'NONE',  ( -0.7874015748031496509, 0.3353269257421728211, -0.2226617707802535651 ) ) ;
#27123=CARTESIAN_POINT ( 'NONE',  ( -0.7434700980050996666, 0.9227202650006829376, -0.1479787484040391843 ) ) ;
#27161=DIRECTION ( 'NONE',  ( 0.000000000000000000, 7.180547322999998243E-06, 0.9999999999742198442 ) ) ;
#27165=B_SPLINE_SURFACE_WITH_KNOTS ( 'NONE', 3, 3, ( 
 ( #22972, #1084, #24931, #7999, #9680 ),
 ( #7858, #1351, #22682, #16602, #3308 ),
 ( #5884, #14512, #23114, #9528, #18128 ),
 ( #26773, #11950, #18281, #7419, #16050 ) ),
 .UNSPECIFIED., .F., .F., .F.,
 ( 4, 4 ),
 ( 4, 1, 4 ),
 ( -0.5999999999999999778, 0.5999999999999999778 ),
 ( -0.003999999999996999879, 1.076708669088524140, 1.887240170904915137 ),
 .UNSPECIFIED. ) ;
#27166=DIRECTION ( 'NONE',  ( -1.000000000000000000, 0.000000000000000000, 0.000000000000000000 ) ) ;
#27178=CARTESIAN_POINT ( 'NONE',  ( 0.3976891862754212137, 1.133679329692560245, -0.4395307839725697274 ) ) ;
#27187=CARTESIAN_POINT ( 'NONE',  ( 0.4898768902087983768, -1.356024015748031595E-16, -0.2362204724409449064 ) ) ;
#27199=CARTESIAN_POINT ( 'NONE',  ( -0.4473595089310440920, -0.7616466953483976843, -0.01204780428933531489 ) ) ;
#27221=CARTESIAN_POINT ( 'NONE',  ( -0.3040421205569480145, 1.096420371425407492, -0.7554543140018661340 ) ) ;
#27223=PLANE ( 'NONE',  #21311 ) ;
#27262=CARTESIAN_POINT ( 'NONE',  ( -0.5638041354701026631, -0.3277633461629020917, 0.1938474616169392761 ) ) ;
#27278=ORIENTED_EDGE ( 'NONE', *, *, #2713, .F. ) ;
#27282=ORIENTED_EDGE ( 'NONE', *, *, #24972, .F. ) ;
#27310=CARTESIAN_POINT ( 'NONE',  ( 0.3339160553493882300, 1.214868409966151530, -0.6104964979807637748 ) ) ;
#27337=CARTESIAN_POINT ( 'NONE',  ( -0.3338887748335570560, -1.269220122646561144, -0.8285976369166339062 ) ) ;
#27351=CARTESIAN_POINT ( 'NONE',  ( -0.5145594007491112176, -0.3210976060043693181, -0.3019172820411493707 ) ) ;
#27358=EDGE_LOOP ( 'NONE', ( #19097, #2892, #16189, #25533 ) ) ;
#27371=EDGE_CURVE ( 'NONE', #22748, #20633, #13468, .T. ) ;
#27372=CARTESIAN_POINT ( 'NONE',  ( -0.2602238532265429005, 0.000000000000000000, -0.2362204724409449064 ) ) ;
#27389=EDGE_LOOP ( 'NONE', ( #14794, #15142, #17098, #3745, #5447, #9568, #23975 ) ) ;
#27416=ORIENTED_EDGE ( 'NONE', *, *, #1786, .T. ) ;
#27434=ADVANCED_FACE ( 'NONE', ( #2462 ), #6994, .F. ) ;
#27461=CARTESIAN_POINT ( 'NONE',  ( 0.4898768902087983768, -2.140741338582677483E-16, 0.2362204724409449064 ) ) ;
#27464=( CONVERSION_BASED_UNIT ( 'INCH', #5859 ) LENGTH_UNIT ( ) NAMED_UNIT ( #10311 ) ) ;
#27472=VERTEX_POINT ( 'NONE', #7689 ) ;
#27480=CARTESIAN_POINT ( 'NONE',  ( -0.5439522672647024715, -0.3016216585743382028, -0.1264851098546873887 ) ) ;
#27491=ORIENTED_EDGE ( 'NONE', *, *, #26541, .F. ) ;
#27526=ORIENTED_EDGE ( 'NONE', *, *, #10164, .F. ) ;
#27554=CARTESIAN_POINT ( 'NONE',  ( -0.5988895145664465680, -0.2041512096132067910, 0.2199573444130424604 ) ) ;
#27597=CARTESIAN_POINT ( 'NONE',  ( -0.7874015748031496509, 0.000000000000000000, -1.052618110236220428 ) ) ;
#27616=CARTESIAN_POINT ( 'NONE',  ( -0.2490711204941346568, 1.208528701367826752, -0.6047752023237676910 ) ) ;
#27622=CARTESIAN_POINT ( 'NONE',  ( -0.6002615430280354714, -0.1506498012739275749, -0.09040378142097618697 ) ) ;
#27636=CARTESIAN_POINT ( 'NONE',  ( -0.5439122934449801550, -0.2529464855333863893, -0.2763027211839643171 ) ) ;
#27658=CARTESIAN_POINT ( 'NONE',  ( -0.6116756676109479374, 0.4474965194255770551, -0.3672460818887063327 ) ) ;
#27686=DIRECTION ( 'NONE',  ( 0.000000000000000000, 7.180547321999995381E-06, -0.9999999999742197332 ) ) ;
#27688=CARTESIAN_POINT ( 'NONE',  ( -0.4331766658145966287, -0.8171300860253869480, -0.05592082628871295619 ) ) ;
#27694=ORIENTED_EDGE ( 'NONE', *, *, #14827, .F. ) ;
#27762=CARTESIAN_POINT ( 'NONE',  ( -0.5833277509429386498, -0.2269466161323728526, 0.05590316927886188753 ) ) ;
#27770=CARTESIAN_POINT ( 'NONE',  ( -0.1361267291514174083, -0.2631590568957330456, 0.2159117096782867951 ) ) ;
#27775=CARTESIAN_POINT ( 'NONE',  ( -0.5618798588062663413, -0.2119744112645649270, -0.2642172244137618309 ) ) ;
#27819=CARTESIAN_POINT ( 'NONE',  ( 0.4895462770359960136, 0.7878044190915924894, -0.4800777499787165503 ) ) ;
#27829=CARTESIAN_POINT ( 'NONE',  ( -0.5646648215863662168, -0.3246897230469174001, 0.1946523111621117075 ) ) ;
#27839=EDGE_CURVE ( 'NONE', #25818, #6360, #3776, .T. ) ;
#27880=CARTESIAN_POINT ( 'NONE',  ( 0.7874015748031496509, -7.558374153346456878E-06, -2.105236220445303008 ) ) ;
ENDSEC;
END-ISO-10303-21;
